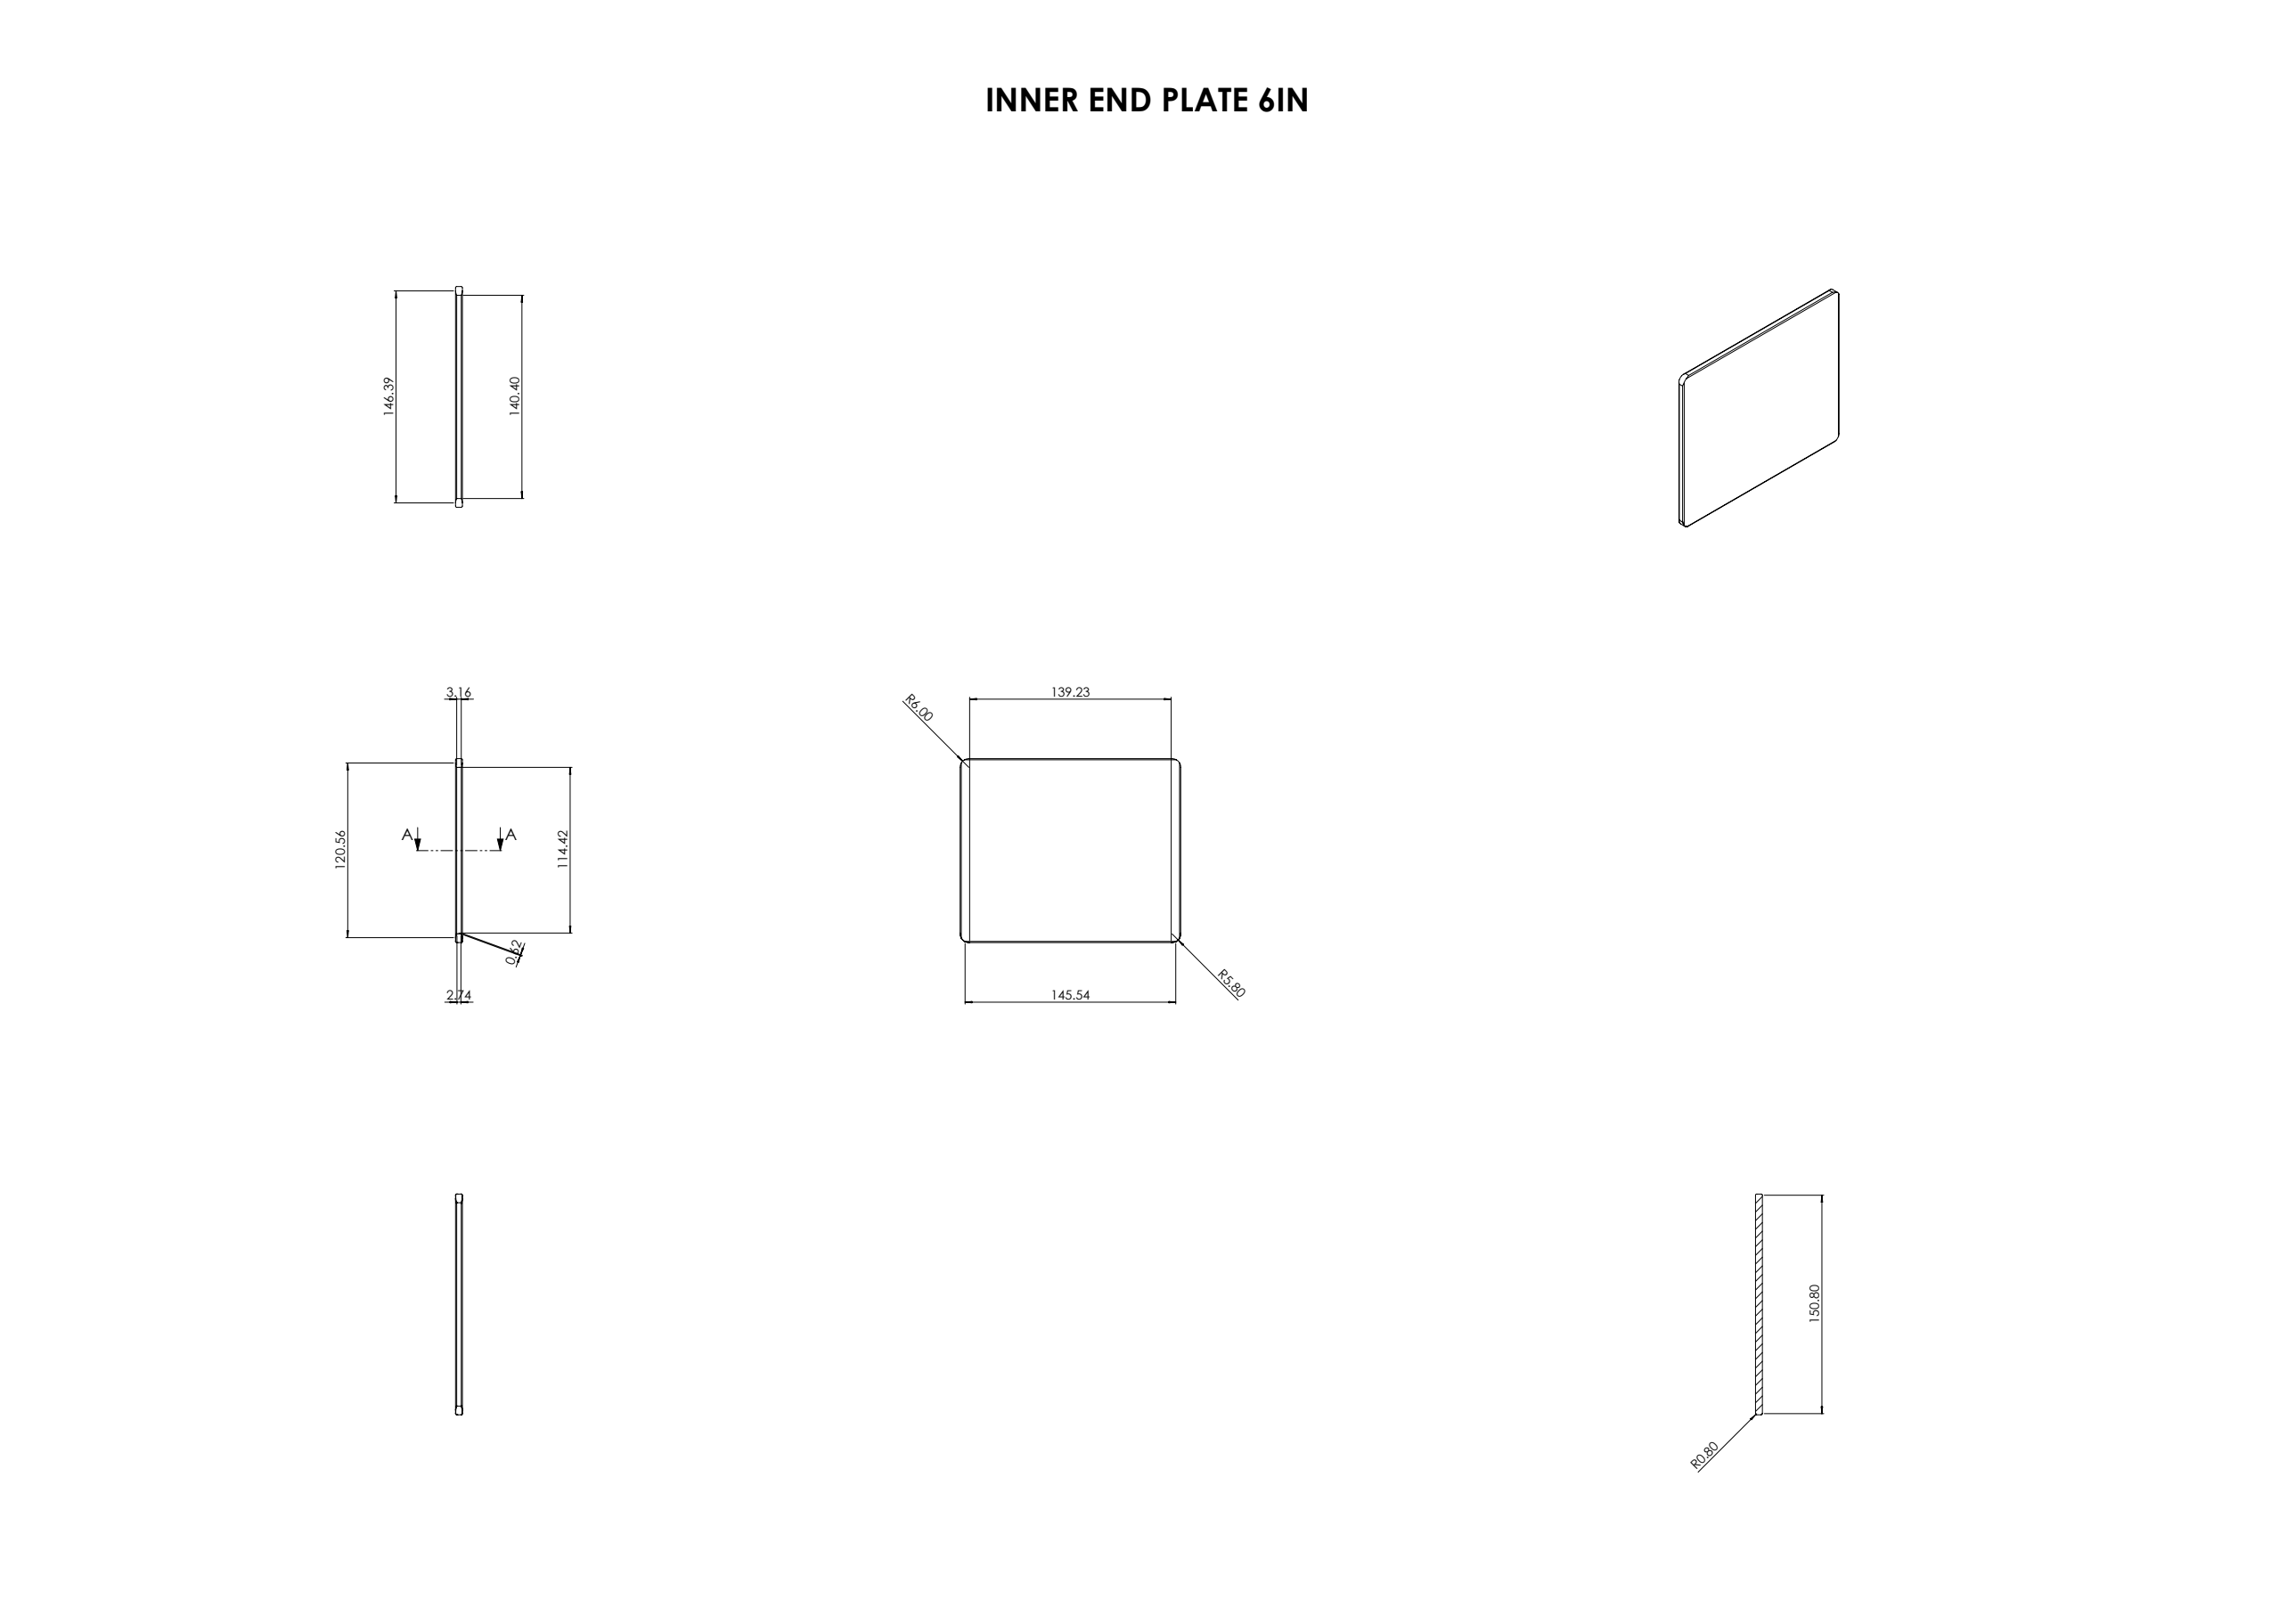
ISO-10303-21;
HEADER;
/* Generated by software containing ST-Developer
 * from STEP Tools, Inc. (www.steptools.com) 
 */

FILE_DESCRIPTION(
/* description */ (''),
/* implementation_level */ '2;1');

FILE_NAME(
/* name */ '06_Inner_End_Plate_6in.step',
/* time_stamp */ '2026-10-25T01:30:15-07:00',
/* author */ (''),
/* organization */ (''),
/* preprocessor_version */ 'ST-DEVELOPER v20.2',
/* originating_system */ 'Autodesk Translation Framework v15.15.0.0',
/* authorisation */ '');

FILE_SCHEMA (('AUTOMOTIVE_DESIGN { 1 0 10303 214 3 1 1 }'));
ENDSEC;

DATA;
#10=MECHANICAL_DESIGN_GEOMETRIC_PRESENTATION_REPRESENTATION('',(#568),#32309);
#192=B_SPLINE_CURVE_WITH_KNOTS('',3,(#22664,#22665,#22666,#22667,#22668,
#22669,#22670,#22671,#22672,#22673,#22674,#22675,#22676,#22677,#22678,#22679,
#22680,#22681,#22682,#22683,#22684,#22685,#22686,#22687,#22688,#22689,#22690,
#22691,#22692,#22693,#22694,#22695,#22696,#22697,#22698,#22699,#22700,#22701,
#22702,#22703,#22704,#22705,#22706,#22707,#22708,#22709,#22710,#22711,#22712,
#22713,#22714,#22715,#22716,#22717,#22718,#22719,#22720,#22721,#22722,#22723,
#22724,#22725,#22726,#22727,#22728,#22729,#22730,#22731,#22732,#22733,#22734,
#22735,#22736,#22737,#22738,#22739,#22740,#22741,#22742,#22743,#22744,#22745),
 .UNSPECIFIED.,.F.,.F.,(4,3,3,3,3,3,3,3,3,3,3,3,3,3,3,3,3,3,3,3,3,3,3,3,
3,3,3,4),(0.,0.0295705059221788,0.060515948666938,0.0926038162611793,0.126139587094163,
0.161619668951817,0.19997110704497,0.243460414557959,0.310976439008441,
0.354040411570413,0.394412885847263,0.429686039983613,0.462833624459996,
0.494651028940637,0.527129557033639,0.560643519237532,0.596019929716605,
0.634095033607031,0.676984117127751,0.757738087845813,0.799051738230702,
0.836280906722732,0.871099048170047,0.903485294449899,0.934889313351429,
0.965468174714213,0.9950913281628,1.),.UNSPECIFIED.);
#193=B_SPLINE_CURVE_WITH_KNOTS('',3,(#22747,#22748,#22749,#22750),
 .UNSPECIFIED.,.F.,.F.,(4,4),(-1.,0.),.UNSPECIFIED.);
#194=B_SPLINE_CURVE_WITH_KNOTS('',3,(#22752,#22753,#22754,#22755,#22756,
#22757,#22758,#22759,#22760,#22761,#22762,#22763,#22764,#22765,#22766,#22767,
#22768,#22769,#22770,#22771,#22772,#22773,#22774,#22775,#22776,#22777,#22778,
#22779,#22780,#22781,#22782,#22783,#22784,#22785,#22786,#22787,#22788,#22789,
#22790,#22791,#22792,#22793,#22794,#22795,#22796,#22797,#22798,#22799,#22800,
#22801,#22802,#22803),.UNSPECIFIED.,.F.,.F.,(4,3,3,3,3,3,3,3,3,3,3,3,3,
3,3,3,3,4),(0.,0.0499444622912523,0.102213229602865,0.161337747228745,0.226027789144595,
0.322774315501521,0.388018395848048,0.444871194111793,0.498045969161039,
0.55130803854745,0.608971254047864,0.676370635210691,0.757277976408018,
0.819640075218638,0.876287936111095,0.929442920609184,0.979183148027167,
1.),.UNSPECIFIED.);
#195=B_SPLINE_CURVE_WITH_KNOTS('',3,(#22843,#22844,#22845,#22846,#22847,
#22848,#22849,#22850,#22851,#22852,#22853,#22854,#22855,#22856,#22857,#22858,
#22859,#22860,#22861,#22862,#22863,#22864,#22865,#22866,#22867,#22868,#22869,
#22870,#22871,#22872,#22873,#22874,#22875,#22876,#22877,#22878,#22879,#22880,
#22881,#22882,#22883,#22884,#22885,#22886,#22887,#22888,#22889,#22890,#22891,
#22892,#22893,#22894),.UNSPECIFIED.,.F.,.F.,(4,3,3,3,3,3,3,3,3,3,3,3,3,
3,3,3,3,4),(0.,0.0499441826810774,0.102212661913948,0.161336812389012,0.22602629684231,
0.322773009737021,0.388016976561433,0.444869601982627,0.498043895325567,
0.551305755159732,0.608968423870093,0.676366592453384,0.757274944340038,
0.819637084908965,0.876284880238144,0.929439762109144,0.979179823244059,
1.),.UNSPECIFIED.);
#196=B_SPLINE_CURVE_WITH_KNOTS('',3,(#22896,#22897,#22898,#22899),
 .UNSPECIFIED.,.F.,.F.,(4,4),(0.,1.),.UNSPECIFIED.);
#197=B_SPLINE_CURVE_WITH_KNOTS('',3,(#22901,#22902,#22903,#22904,#22905,
#22906,#22907,#22908,#22909,#22910,#22911,#22912,#22913,#22914,#22915,#22916,
#22917,#22918,#22919,#22920,#22921,#22922,#22923,#22924,#22925,#22926,#22927,
#22928,#22929,#22930,#22931,#22932,#22933,#22934,#22935,#22936,#22937,#22938,
#22939,#22940,#22941,#22942,#22943,#22944,#22945,#22946,#22947,#22948,#22949,
#22950,#22951,#22952,#22953,#22954,#22955,#22956,#22957,#22958,#22959,#22960,
#22961,#22962,#22963,#22964,#22965,#22966,#22967,#22968,#22969,#22970,#22971,
#22972,#22973,#22974,#22975,#22976,#22977,#22978,#22979,#22980,#22981,#22982),
 .UNSPECIFIED.,.F.,.F.,(4,3,3,3,3,3,3,3,3,3,3,3,3,3,3,3,3,3,3,3,3,3,3,3,
3,3,3,4),(0.,0.0295773881145616,0.060530416968692,0.0926266479896254,0.126171922797507,
0.161663359409179,0.200029752326511,0.243548698803929,0.310961877352299,
0.35402676001778,0.394400087516669,0.429679984519188,0.462839399605369,
0.494661354038637,0.527132669662275,0.560640871657354,0.59601115409547,
0.63407950773062,0.676959315385358,0.757719486539019,0.799022960212248,
0.836244253893979,0.871055469575998,0.903435210203506,0.934833075272902,
0.965406057017476,0.995023142061764,1.),.UNSPECIFIED.);
#198=B_SPLINE_CURVE_WITH_KNOTS('',3,(#23001,#23002,#23003,#23004),
 .UNSPECIFIED.,.F.,.F.,(4,4),(9.99629094513139E-5,0.273153287835102),
 .UNSPECIFIED.);
#199=B_SPLINE_CURVE_WITH_KNOTS('',3,(#23007,#23008,#23009,#23010),
 .UNSPECIFIED.,.F.,.F.,(4,4),(-0.273153287835102,-9.99629094513139E-5),
 .UNSPECIFIED.);
#200=B_SPLINE_CURVE_WITH_KNOTS('',3,(#23036,#23037,#23038,#23039),
 .UNSPECIFIED.,.F.,.F.,(4,4),(-0.310482170393536,-0.273153287835088),
 .UNSPECIFIED.);
#201=B_SPLINE_CURVE_WITH_KNOTS('',3,(#23040,#23041,#23042,#23043),
 .UNSPECIFIED.,.F.,.F.,(4,4),(0.273153287835088,0.310482170393536),
 .UNSPECIFIED.);
#202=B_SPLINE_CURVE_WITH_KNOTS('',3,(#23069,#23070,#23071,#23072,#23073,
#23074),.UNSPECIFIED.,.F.,.F.,(4,2,4),(-0.954291288267866,-0.799150016166134,
-0.681237813527804),.UNSPECIFIED.);
#203=B_SPLINE_CURVE_WITH_KNOTS('',3,(#23077,#23078,#23079,#23080,#23081,
#23082),.UNSPECIFIED.,.F.,.F.,(4,2,4),(0.681237813527804,0.799150016166134,
0.954291288267866),.UNSPECIFIED.);
#204=B_SPLINE_CURVE_WITH_KNOTS('',3,(#23099,#23100,#23101,#23102),
 .UNSPECIFIED.,.F.,.F.,(4,4),(-0.681237813527818,-0.643908930969367),
 .UNSPECIFIED.);
#205=B_SPLINE_CURVE_WITH_KNOTS('',3,(#23103,#23104,#23105,#23106),
 .UNSPECIFIED.,.F.,.F.,(4,4),(0.643908930969367,0.681237813527818),
 .UNSPECIFIED.);
#206=B_SPLINE_CURVE_WITH_KNOTS('',3,(#23111,#23112,#23113,#23114,#23115,
#23116),.UNSPECIFIED.,.F.,.F.,(4,2,4),(0.,0.155241085196768,0.310482170393536),
 .UNSPECIFIED.);
#207=B_SPLINE_CURVE_WITH_KNOTS('',3,(#23130,#23131,#23132,#23133,#23134,
#23135,#23136,#23137,#23138,#23139,#23140,#23141,#23142,#23143,#23144,#23145,
#23146,#23147,#23148,#23149,#23150,#23151,#23152,#23153,#23154,#23155,#23156,
#23157,#23158,#23159,#23160,#23161,#23162,#23163,#23164,#23165,#23166,#23167,
#23168,#23169,#23170,#23171,#23172,#23173,#23174,#23175,#23176,#23177,#23178,
#23179,#23180,#23181),.UNSPECIFIED.,.F.,.F.,(4,3,3,3,3,3,3,3,3,3,3,3,3,
3,3,3,3,4),(0.,0.0499444619143997,0.102213228836067,0.161337745961679,0.226027787112555,
0.322774313723485,0.388018393939231,0.444871191980803,0.498045966386616,
0.551308035462484,0.608971250191218,0.676370629650621,0.757277972237966,
0.819640071099801,0.876287931893757,0.929442916241627,0.979183143421037,
1.),.UNSPECIFIED.);
#208=B_SPLINE_CURVE_WITH_KNOTS('',3,(#23183,#23184,#23185,#23186),
 .UNSPECIFIED.,.F.,.F.,(4,4),(0.681229980645393,0.954283455385461),
 .UNSPECIFIED.);
#209=B_SPLINE_CURVE_WITH_KNOTS('',3,(#23188,#23189,#23190,#23191),
 .UNSPECIFIED.,.F.,.F.,(4,4),(0.64390109808696,0.681229980645406),
 .UNSPECIFIED.);
#210=B_SPLINE_CURVE_WITH_KNOTS('',3,(#23195,#23196,#23197,#23198),
 .UNSPECIFIED.,.F.,.F.,(4,4),(0.273153287835084,0.310482170393536),
 .UNSPECIFIED.);
#211=B_SPLINE_CURVE_WITH_KNOTS('',3,(#23200,#23201,#23202,#23203),
 .UNSPECIFIED.,.F.,.F.,(4,4),(9.9962909451316E-5,0.273153287835098),
 .UNSPECIFIED.);
#212=B_SPLINE_CURVE_WITH_KNOTS('',3,(#23204,#23205,#23206,#23207,#23208,
#23209,#23210,#23211,#23212,#23213,#23214,#23215,#23216,#23217,#23218,#23219,
#23220,#23221,#23222,#23223,#23224,#23225,#23226,#23227,#23228,#23229,#23230,
#23231,#23232,#23233,#23234,#23235,#23236,#23237,#23238,#23239,#23240,#23241,
#23242,#23243,#23244,#23245,#23246,#23247,#23248,#23249,#23250,#23251,#23252,
#23253,#23254,#23255),.UNSPECIFIED.,.F.,.F.,(4,3,3,3,3,3,3,3,3,3,3,3,3,
3,3,3,3,4),(0.,0.0499441833890994,0.102212663354842,0.161336814770156,0.226026300658892,
0.322773013076531,0.388016980146127,0.44486960598537,0.498043900535783,
0.551305760953592,0.608968431113942,0.676366602895863,0.757274952171898,
0.819637092644225,0.876284888158664,0.929439770311992,0.979179831894635,
1.),.UNSPECIFIED.);
#213=B_SPLINE_CURVE_WITH_KNOTS('',3,(#23278,#23279,#23280,#23281,#23282,
#23283,#23284,#23285,#23286,#23287,#23288,#23289,#23290,#23291,#23292,#23293,
#23294,#23295,#23296,#23297,#23298,#23299,#23300,#23301,#23302,#23303,#23304,
#23305,#23306,#23307,#23308,#23309,#23310,#23311,#23312,#23313,#23314,#23315,
#23316,#23317,#23318,#23319,#23320,#23321,#23322,#23323,#23324,#23325,#23326,
#23327,#23328,#23329,#23330,#23331,#23332,#23333,#23334,#23335,#23336,#23337,
#23338,#23339,#23340,#23341,#23342,#23343,#23344,#23345,#23346,#23347,#23348,
#23349,#23350,#23351,#23352,#23353,#23354,#23355,#23356,#23357,#23358,#23359),
 .UNSPECIFIED.,.F.,.F.,(4,3,3,3,3,3,3,3,3,3,3,3,3,3,3,3,3,3,3,3,3,3,3,3,
3,3,3,4),(0.,0.0295705059449982,0.0605159487132195,0.0926038163323903,0.126139587195106,
0.161619669086869,0.199971107221821,0.243460414815925,0.310976439628805,
0.354040412152005,0.394412886392504,0.42968604051999,0.462833625082738,
0.494651029536218,0.527129557597107,0.56064351985676,0.596019930404549,
0.634095034387078,0.676984118085056,0.757738088563792,0.79905173888368,
0.836280907354532,0.871099048793566,0.903485295079146,0.934889313990762,
0.965468175362615,0.99509132882554,1.),.UNSPECIFIED.);
#214=B_SPLINE_CURVE_WITH_KNOTS('',3,(#23361,#23362,#23363,#23364),
 .UNSPECIFIED.,.F.,.F.,(4,4),(-1.,0.),.UNSPECIFIED.);
#215=B_SPLINE_CURVE_WITH_KNOTS('',3,(#23366,#23367,#23368,#23369,#23370,
#23371,#23372,#23373,#23374,#23375,#23376,#23377,#23378,#23379,#23380,#23381,
#23382,#23383,#23384,#23385,#23386,#23387,#23388,#23389,#23390,#23391,#23392,
#23393,#23394,#23395,#23396,#23397,#23398,#23399,#23400,#23401,#23402,#23403,
#23404,#23405,#23406,#23407,#23408,#23409,#23410,#23411,#23412,#23413,#23414,
#23415,#23416,#23417),.UNSPECIFIED.,.F.,.F.,(4,3,3,3,3,3,3,3,3,3,3,3,3,
3,3,3,3,4),(0.,0.0499444620030573,0.102213229017714,0.161337746261311,0.226027787592192,
0.322774314143168,0.388018394389041,0.444871192483061,0.498045967040621,
0.551308036189455,0.608971251099731,0.676370630959906,0.757277973219929,
0.819640072069571,0.876287932886441,0.929442917270342,0.979183144505862,
1.),.UNSPECIFIED.);
#216=B_SPLINE_CURVE_WITH_KNOTS('',3,(#23457,#23458,#23459,#23460,#23461,
#23462,#23463,#23464,#23465,#23466,#23467,#23468,#23469,#23470,#23471,#23472,
#23473,#23474,#23475,#23476,#23477,#23478,#23479,#23480,#23481,#23482,#23483,
#23484,#23485,#23486,#23487,#23488,#23489,#23490,#23491,#23492,#23493,#23494,
#23495,#23496,#23497,#23498,#23499,#23500,#23501,#23502,#23503,#23504,#23505,
#23506,#23507,#23508),.UNSPECIFIED.,.F.,.F.,(4,3,3,3,3,3,3,3,3,3,3,3,3,
3,3,3,3,4),(0.,0.0499441826811105,0.102212661914011,0.161336812389129,0.226026296842565,
0.322773009737244,0.388016976561584,0.444869601982792,0.498043895325763,
0.551305755159944,0.608968423870338,0.676366592453702,0.757274944340276,
0.819637084909205,0.876284880238396,0.929439762109376,0.979179823244325,
1.),.UNSPECIFIED.);
#217=B_SPLINE_CURVE_WITH_KNOTS('',3,(#23510,#23511,#23512,#23513),
 .UNSPECIFIED.,.F.,.F.,(4,4),(0.,1.),.UNSPECIFIED.);
#218=B_SPLINE_CURVE_WITH_KNOTS('',3,(#23515,#23516,#23517,#23518,#23519,
#23520,#23521,#23522,#23523,#23524,#23525,#23526,#23527,#23528,#23529,#23530,
#23531,#23532,#23533,#23534,#23535,#23536,#23537,#23538,#23539,#23540,#23541,
#23542,#23543,#23544,#23545,#23546,#23547,#23548,#23549,#23550,#23551,#23552,
#23553,#23554,#23555,#23556,#23557,#23558,#23559,#23560,#23561,#23562,#23563,
#23564,#23565,#23566,#23567,#23568,#23569,#23570,#23571,#23572,#23573,#23574,
#23575,#23576,#23577,#23578,#23579,#23580,#23581,#23582,#23583,#23584,#23585,
#23586,#23587,#23588,#23589,#23590,#23591,#23592,#23593,#23594,#23595,#23596),
 .UNSPECIFIED.,.F.,.F.,(4,3,3,3,3,3,3,3,3,3,3,3,3,3,3,3,3,3,3,3,3,3,3,3,
3,3,3,4),(0.,0.0295773881131102,0.0605304169672427,0.0926266479882803,0.126171922795967,
0.161663359407986,0.20002975232552,0.243548698802509,0.31096187735372,0.354026760019112,
0.394400087517918,0.429679984520021,0.462839399606215,0.494661354039968,
0.527132669663605,0.560640871658796,0.596011154096698,0.63407950773218,
0.676959315385293,0.75771948653897,0.799022960211628,0.836244253893244,
0.871055469575763,0.903435210203173,0.934833075272608,0.965406057016351,
0.995023142060179,1.),.UNSPECIFIED.);
#219=B_SPLINE_CURVE_WITH_KNOTS('',3,(#23615,#23616,#23617,#23618),
 .UNSPECIFIED.,.F.,.F.,(4,4),(9.99629094513149E-5,0.273153287835104),
 .UNSPECIFIED.);
#220=B_SPLINE_CURVE_WITH_KNOTS('',3,(#23621,#23622,#23623,#23624),
 .UNSPECIFIED.,.F.,.F.,(4,4),(-0.273153287835104,-9.99629094513149E-5),
 .UNSPECIFIED.);
#221=B_SPLINE_CURVE_WITH_KNOTS('',3,(#23650,#23651,#23652,#23653),
 .UNSPECIFIED.,.F.,.F.,(4,4),(-0.310482170393536,-0.273153287835091),
 .UNSPECIFIED.);
#222=B_SPLINE_CURVE_WITH_KNOTS('',3,(#23654,#23655,#23656,#23657),
 .UNSPECIFIED.,.F.,.F.,(4,4),(0.273153287835091,0.310482170393536),
 .UNSPECIFIED.);
#223=B_SPLINE_CURVE_WITH_KNOTS('',3,(#23675,#23676,#23677,#23678),
 .UNSPECIFIED.,.F.,.F.,(4,4),(-0.954283455385459,-0.681229980645392),
 .UNSPECIFIED.);
#224=B_SPLINE_CURVE_WITH_KNOTS('',3,(#23681,#23682,#23683,#23684),
 .UNSPECIFIED.,.F.,.F.,(4,4),(0.681229980645392,0.954283455385459),
 .UNSPECIFIED.);
#225=B_SPLINE_CURVE_WITH_KNOTS('',3,(#23701,#23702,#23703,#23704),
 .UNSPECIFIED.,.F.,.F.,(4,4),(-0.681229980645406,-0.643901098086959),
 .UNSPECIFIED.);
#226=B_SPLINE_CURVE_WITH_KNOTS('',3,(#23705,#23706,#23707,#23708),
 .UNSPECIFIED.,.F.,.F.,(4,4),(0.643901098086959,0.681229980645406),
 .UNSPECIFIED.);
#227=B_SPLINE_CURVE_WITH_KNOTS('',3,(#23722,#23723,#23724,#23725,#23726,
#23727),.UNSPECIFIED.,.F.,.F.,(4,2,4),(0.643901098086957,0.799142183283726,
0.954383268480494),.UNSPECIFIED.);
#228=B_SPLINE_CURVE_WITH_KNOTS('',3,(#23757,#23758,#23759,#23760,#23761,
#23762,#23763,#23764,#23765,#23766,#23767,#23768,#23769,#23770,#23771,#23772,
#23773,#23774,#23775,#23776,#23777,#23778,#23779,#23780,#23781,#23782,#23783,
#23784,#23785,#23786,#23787,#23788,#23789,#23790,#23791,#23792,#23793,#23794,
#23795,#23796,#23797,#23798,#23799,#23800,#23801,#23802,#23803,#23804,#23805,
#23806,#23807,#23808,#23809,#23810,#23811,#23812,#23813,#23814,#23815,#23816,
#23817,#23818,#23819,#23820,#23821,#23822,#23823,#23824,#23825,#23826,#23827,
#23828,#23829,#23830,#23831,#23832,#23833,#23834,#23835,#23836,#23837,#23838),
 .UNSPECIFIED.,.F.,.F.,(4,3,3,3,3,3,3,3,3,3,3,3,3,3,3,3,3,3,3,3,3,3,3,3,
3,3,3,4),(0.,0.0295705059512633,0.0605159487271851,0.0926038163550416,0.126139587225611,
0.161619669126796,0.199971107275455,0.243460414898968,0.31097643981881,
0.354040412330134,0.394412886559501,0.429686040686443,0.46283362527423,
0.494651029717672,0.527129557769278,0.560643520045596,0.596019930614712,
0.634095034624437,0.676984118378702,0.757738088784027,0.799051739082071,
0.836280907545797,0.871099048983326,0.903485295270873,0.934889314183803,
0.965468175561812,0.995091329030122,1.),.UNSPECIFIED.);
#229=B_SPLINE_CURVE_WITH_KNOTS('',3,(#23839,#23840,#23841,#23842),
 .UNSPECIFIED.,.F.,.F.,(4,4),(-1.,0.),.UNSPECIFIED.);
#230=B_SPLINE_CURVE_WITH_KNOTS('',3,(#23881,#23882,#23883,#23884),
 .UNSPECIFIED.,.F.,.F.,(4,4),(0.,1.),.UNSPECIFIED.);
#231=B_SPLINE_CURVE_WITH_KNOTS('',3,(#23885,#23886,#23887,#23888,#23889,
#23890,#23891,#23892,#23893,#23894,#23895,#23896,#23897,#23898,#23899,#23900,
#23901,#23902,#23903,#23904,#23905,#23906,#23907,#23908,#23909,#23910,#23911,
#23912,#23913,#23914,#23915,#23916,#23917,#23918,#23919,#23920,#23921,#23922,
#23923,#23924,#23925,#23926,#23927,#23928,#23929,#23930,#23931,#23932,#23933,
#23934,#23935,#23936,#23937,#23938,#23939,#23940,#23941,#23942,#23943,#23944,
#23945,#23946,#23947,#23948,#23949,#23950,#23951,#23952,#23953,#23954,#23955,
#23956,#23957,#23958,#23959,#23960,#23961,#23962,#23963,#23964,#23965,#23966),
 .UNSPECIFIED.,.F.,.F.,(4,3,3,3,3,3,3,3,3,3,3,3,3,3,3,3,3,3,3,3,3,3,3,3,
3,3,3,4),(0.,0.0295773880524302,0.0605304168410243,0.092626647792498,0.126171922525243,
0.161663359050634,0.200029751864124,0.24354869819935,0.31096188049952,0.3540267629683,
0.394400090282781,0.429679987033957,0.462839402284777,0.494661356438073,
0.527132671762529,0.560640873794645,0.59601115629688,0.634079510052112,
0.676959318040989,0.757719488530741,0.799022961866045,0.836244255350966,
0.871055470885213,0.903435211410382,0.934833076388468,0.965406058048494,
0.995023143024151,1.),.UNSPECIFIED.);
#232=B_SPLINE_CURVE_WITH_KNOTS('',3,(#23985,#23986,#23987,#23988),
 .UNSPECIFIED.,.F.,.F.,(4,4),(-0.273153287835098,-9.9962909451316E-5),
 .UNSPECIFIED.);
#233=B_SPLINE_CURVE_WITH_KNOTS('',3,(#24011,#24012,#24013,#24014),
 .UNSPECIFIED.,.F.,.F.,(4,4),(-0.310482170393536,-0.273153287835084),
 .UNSPECIFIED.);
#234=B_SPLINE_CURVE_WITH_KNOTS('',3,(#24032,#24033,#24034,#24035),
 .UNSPECIFIED.,.F.,.F.,(4,4),(-0.954283455385461,-0.681229980645393),
 .UNSPECIFIED.);
#235=B_SPLINE_CURVE_WITH_KNOTS('',3,(#24053,#24054,#24055,#24056),
 .UNSPECIFIED.,.F.,.F.,(4,4),(-0.681229980645406,-0.64390109808696),
 .UNSPECIFIED.);
#236=B_SPLINE_CURVE_WITH_KNOTS('',3,(#24061,#24062,#24063,#24064,#24065,
#24066,#24067,#24068,#24069,#24070,#24071,#24072,#24073,#24074,#24075,#24076,
#24077,#24078,#24079,#24080,#24081,#24082,#24083,#24084,#24085,#24086,#24087,
#24088,#24089,#24090,#24091,#24092,#24093,#24094,#24095,#24096,#24097,#24098,
#24099,#24100,#24101,#24102,#24103,#24104,#24105,#24106,#24107,#24108,#24109,
#24110,#24111,#24112,#24113,#24114,#24115,#24116,#24117,#24118,#24119,#24120,
#24121,#24122,#24123,#24124,#24125,#24126,#24127,#24128,#24129,#24130,#24131,
#24132,#24133,#24134,#24135,#24136,#24137,#24138,#24139,#24140,#24141,#24142),
 .UNSPECIFIED.,.F.,.F.,(4,3,3,3,3,3,3,3,3,3,3,3,3,3,3,3,3,3,3,3,3,3,3,3,
3,3,3,4),(0.,0.029577388096564,0.0605304169342327,0.092626647938075,0.126171922726201,
0.161663359317722,0.200029752207105,0.243548698650945,0.310961878143349,
0.354026760759389,0.394400088211927,0.42967998515154,0.462839400279756,
0.49466135464192,0.527132670190963,0.560640872195637,0.596011154650127,
0.634079508317272,0.676959316055784,0.757719487041838,0.799022960628449,
0.836244254262571,0.871055469905186,0.903435210506207,0.934833075552335,
0.965406057277606,0.995023142305148,1.),.UNSPECIFIED.);
#237=B_SPLINE_CURVE_WITH_KNOTS('',3,(#24144,#24145,#24146,#24147),
 .UNSPECIFIED.,.F.,.F.,(4,4),(-0.273153287835103,-9.99629094513129E-5),
 .UNSPECIFIED.);
#238=B_SPLINE_CURVE_WITH_KNOTS('',3,(#24175,#24176,#24177,#24178,#24179,
#24180,#24181,#24182,#24183,#24184,#24185,#24186,#24187,#24188,#24189,#24190,
#24191,#24192,#24193,#24194,#24195,#24196,#24197,#24198,#24199,#24200,#24201,
#24202,#24203,#24204,#24205,#24206,#24207,#24208,#24209,#24210,#24211,#24212,
#24213,#24214,#24215,#24216,#24217,#24218,#24219,#24220,#24221,#24222,#24223,
#24224,#24225,#24226,#24227,#24228,#24229,#24230,#24231,#24232,#24233,#24234,
#24235,#24236,#24237,#24238,#24239,#24240,#24241,#24242,#24243,#24244,#24245,
#24246,#24247,#24248,#24249,#24250,#24251,#24252,#24253,#24254,#24255,#24256),
 .UNSPECIFIED.,.F.,.F.,(4,3,3,3,3,3,3,3,3,3,3,3,3,3,3,3,3,3,3,3,3,3,3,3,
3,3,3,4),(0.,0.0295705059230571,0.0605159486675307,0.0926038162612098,0.126139587094081,
0.161619668951887,0.199971107044072,0.243460414557264,0.310976439007079,
0.354040411569137,0.394412885846066,0.429686039982072,0.462833624458263,
0.494651028937512,0.527129557030697,0.560643519234331,0.596019929713393,
0.634095033602269,0.676984117126932,0.757738087845199,0.799051738231756,
0.836280906723594,0.871099048170336,0.903485294450174,0.934889313352345,
0.965468174717861,0.99509132816655,1.),.UNSPECIFIED.);
#239=B_SPLINE_CURVE_WITH_KNOTS('',3,(#24258,#24259,#24260,#24261),
 .UNSPECIFIED.,.F.,.F.,(4,4),(-1.,0.),.UNSPECIFIED.);
#240=B_SPLINE_CURVE_WITH_KNOTS('',3,(#24262,#24263,#24264,#24265,#24266,
#24267,#24268,#24269,#24270,#24271,#24272,#24273,#24274,#24275,#24276,#24277,
#24278,#24279,#24280,#24281,#24282,#24283,#24284,#24285,#24286,#24287,#24288,
#24289,#24290,#24291,#24292,#24293,#24294,#24295,#24296,#24297,#24298,#24299,
#24300,#24301,#24302,#24303,#24304,#24305,#24306,#24307,#24308,#24309,#24310,
#24311,#24312,#24313),.UNSPECIFIED.,.F.,.F.,(4,3,3,3,3,3,3,3,3,3,3,3,3,
3,3,3,3,4),(0.,0.0499444622913127,0.102213229603,0.161337747229144,0.226027789144532,
0.322774315501466,0.388018395848148,0.444871194112166,0.498045969161075,
0.551308038547837,0.60897125404869,0.676370635211665,0.757277976408749,
0.81964007521899,0.876287936111462,0.92944292060967,0.979183148027608,1.),
 .UNSPECIFIED.);
#241=B_SPLINE_CURVE_WITH_KNOTS('',3,(#24351,#24352,#24353,#24354,#24355,
#24356,#24357,#24358,#24359,#24360,#24361,#24362,#24363,#24364,#24365,#24366,
#24367,#24368,#24369,#24370,#24371,#24372,#24373,#24374,#24375,#24376,#24377,
#24378,#24379,#24380,#24381,#24382,#24383,#24384,#24385,#24386,#24387,#24388,
#24389,#24390,#24391,#24392,#24393,#24394,#24395,#24396,#24397,#24398,#24399,
#24400,#24401,#24402),.UNSPECIFIED.,.F.,.F.,(4,3,3,3,3,3,3,3,3,3,3,3,3,
3,3,3,3,4),(0.,0.0499441828589668,0.102212662275513,0.161336812986304,0.226026297799104,
0.322773010574216,0.388016977460993,0.444869602986684,0.498043896631638,
0.551305756611869,0.608968425686129,0.676366595071555,0.757274946303666,
0.819637086848271,0.876284882223587,0.929439764165566,0.979179825412561,
1.),.UNSPECIFIED.);
#242=B_SPLINE_CURVE_WITH_KNOTS('',3,(#24403,#24404,#24405,#24406),
 .UNSPECIFIED.,.F.,.F.,(4,4),(0.,1.),.UNSPECIFIED.);
#243=B_SPLINE_CURVE_WITH_KNOTS('',3,(#24424,#24425,#24426,#24427),
 .UNSPECIFIED.,.F.,.F.,(4,4),(9.99629094513129E-5,0.273153287835103),
 .UNSPECIFIED.);
#244=B_SPLINE_CURVE_WITH_KNOTS('',3,(#24454,#24455,#24456,#24457),
 .UNSPECIFIED.,.F.,.F.,(4,4),(-0.310482170393537,-0.273153287835089),
 .UNSPECIFIED.);
#245=B_SPLINE_CURVE_WITH_KNOTS('',3,(#24458,#24459,#24460,#24461),
 .UNSPECIFIED.,.F.,.F.,(4,4),(0.273153287835089,0.310482170393537),
 .UNSPECIFIED.);
#246=B_SPLINE_CURVE_WITH_KNOTS('',3,(#24479,#24480,#24481,#24482),
 .UNSPECIFIED.,.F.,.F.,(4,4),(-0.95428345538546,-0.681229980645392),
 .UNSPECIFIED.);
#247=B_SPLINE_CURVE_WITH_KNOTS('',3,(#24485,#24486,#24487,#24488),
 .UNSPECIFIED.,.F.,.F.,(4,4),(0.681229980645392,0.95428345538546),
 .UNSPECIFIED.);
#248=B_SPLINE_CURVE_WITH_KNOTS('',3,(#24505,#24506,#24507,#24508),
 .UNSPECIFIED.,.F.,.F.,(4,4),(-0.681229980645405,-0.643901098086959),
 .UNSPECIFIED.);
#249=B_SPLINE_CURVE_WITH_KNOTS('',3,(#24509,#24510,#24511,#24512),
 .UNSPECIFIED.,.F.,.F.,(4,4),(0.643901098086959,0.681229980645405),
 .UNSPECIFIED.);
#250=B_SPLINE_CURVE_WITH_KNOTS('',3,(#24526,#24527,#24528,#24529,#24530,
#24531),.UNSPECIFIED.,.F.,.F.,(4,2,4),(0.,0.155241085196768,0.310482170393536),
 .UNSPECIFIED.);
#251=B_SPLINE_CURVE_WITH_KNOTS('',3,(#24534,#24535,#24536,#24537,#24538,
#24539),.UNSPECIFIED.,.F.,.F.,(4,2,4),(0.,0.155241085196768,0.310482170393535),
 .UNSPECIFIED.);
#252=B_SPLINE_CURVE_WITH_KNOTS('',3,(#24542,#24543,#24544,#24545,#24546,
#24547),.UNSPECIFIED.,.F.,.F.,(4,2,4),(0.643908930969365,0.799150016166132,
0.9543911013629),.UNSPECIFIED.);
#253=B_SPLINE_CURVE_WITH_KNOTS('',3,(#24550,#24551,#24552,#24553,#24554,
#24555),.UNSPECIFIED.,.F.,.F.,(4,2,4),(0.,0.15524108519677,0.310482170393539),
 .UNSPECIFIED.);
#254=B_SPLINE_CURVE_WITH_KNOTS('',3,(#24560,#24561,#24562,#24563,#24564,
#24565),.UNSPECIFIED.,.F.,.F.,(4,2,4),(0.643908930969368,0.799150016166137,
0.954391101362907),.UNSPECIFIED.);
#255=B_SPLINE_CURVE_WITH_KNOTS('',3,(#24566,#24567,#24568,#24569,#24570,
#24571),.UNSPECIFIED.,.F.,.F.,(4,2,4),(0.643908930969366,0.799150016166134,
0.954391101362902),.UNSPECIFIED.);
#447=B_SPLINE_SURFACE_WITH_KNOTS('',3,3,((#22642,#22643,#22644,#22645,#22646),
(#22647,#22648,#22649,#22650,#22651),(#22652,#22653,#22654,#22655,#22656),
(#22657,#22658,#22659,#22660,#22661)),.UNSPECIFIED.,.F.,.F.,.F.,(4,4),(4,
1,4),(0.,1.),(0.,0.571428571428571,1.),.UNSPECIFIED.);
#448=B_SPLINE_SURFACE_WITH_KNOTS('',3,3,((#22805,#22806,#22807,#22808,#22809,
#22810,#22811,#22812,#22813),(#22814,#22815,#22816,#22817,#22818,#22819,
#22820,#22821,#22822),(#22823,#22824,#22825,#22826,#22827,#22828,#22829,
#22830,#22831),(#22832,#22833,#22834,#22835,#22836,#22837,#22838,#22839,
#22840)),.UNSPECIFIED.,.F.,.F.,.F.,(4,4),(4,1,1,1,1,1,4),(0.,1.),(0.,0.214285714285714,
0.357142857142857,0.571428571428571,0.785714285714286,0.857142857142857,
1.),.UNSPECIFIED.);
#449=B_SPLINE_SURFACE_WITH_KNOTS('',3,3,((#22984,#22985,#22986,#22987),
(#22988,#22989,#22990,#22991),(#22992,#22993,#22994,#22995),(#22996,#22997,
#22998,#22999)),.UNSPECIFIED.,.F.,.F.,.F.,(4,4),(4,4),(0.,1.),(9.99629094513139E-5,
0.273153287835102),.UNSPECIFIED.);
#450=B_SPLINE_SURFACE_WITH_KNOTS('',3,3,((#23020,#23021,#23022,#23023),
(#23024,#23025,#23026,#23027),(#23028,#23029,#23030,#23031),(#23032,#23033,
#23034,#23035)),.UNSPECIFIED.,.F.,.F.,.F.,(4,4),(4,4),(0.,1.),(0.273153287835088,
0.310482170393536),.UNSPECIFIED.);
#451=B_SPLINE_SURFACE_WITH_KNOTS('',3,3,((#23044,#23045,#23046,#23047,#23048,
#23049),(#23050,#23051,#23052,#23053,#23054,#23055),(#23056,#23057,#23058,
#23059,#23060,#23061),(#23062,#23063,#23064,#23065,#23066,#23067)),
 .UNSPECIFIED.,.F.,.F.,.F.,(4,4),(4,2,4),(0.,1.),(0.681237813527804,0.799150016166134,
0.954291288267866),.UNSPECIFIED.);
#452=B_SPLINE_SURFACE_WITH_KNOTS('',3,3,((#23083,#23084,#23085,#23086),
(#23087,#23088,#23089,#23090),(#23091,#23092,#23093,#23094),(#23095,#23096,
#23097,#23098)),.UNSPECIFIED.,.F.,.F.,.F.,(4,4),(4,4),(0.,1.),(0.643908930969367,
0.681237813527818),.UNSPECIFIED.);
#453=B_SPLINE_SURFACE_WITH_KNOTS('',3,3,((#23256,#23257,#23258,#23259,#23260),
(#23261,#23262,#23263,#23264,#23265),(#23266,#23267,#23268,#23269,#23270),
(#23271,#23272,#23273,#23274,#23275)),.UNSPECIFIED.,.F.,.F.,.F.,(4,4),(4,
1,4),(0.,1.),(0.,0.571428571428571,1.),.UNSPECIFIED.);
#454=B_SPLINE_SURFACE_WITH_KNOTS('',3,3,((#23419,#23420,#23421,#23422,#23423,
#23424,#23425,#23426,#23427),(#23428,#23429,#23430,#23431,#23432,#23433,
#23434,#23435,#23436),(#23437,#23438,#23439,#23440,#23441,#23442,#23443,
#23444,#23445),(#23446,#23447,#23448,#23449,#23450,#23451,#23452,#23453,
#23454)),.UNSPECIFIED.,.F.,.F.,.F.,(4,4),(4,1,1,1,1,1,4),(0.,1.),(0.,0.214285714285714,
0.357142857142857,0.571428571428571,0.785714285714286,0.857142857142857,
1.),.UNSPECIFIED.);
#455=B_SPLINE_SURFACE_WITH_KNOTS('',3,3,((#23598,#23599,#23600,#23601),
(#23602,#23603,#23604,#23605),(#23606,#23607,#23608,#23609),(#23610,#23611,
#23612,#23613)),.UNSPECIFIED.,.F.,.F.,.F.,(4,4),(4,4),(0.,1.),(9.99629094513149E-5,
0.273153287835104),.UNSPECIFIED.);
#456=B_SPLINE_SURFACE_WITH_KNOTS('',3,3,((#23634,#23635,#23636,#23637),
(#23638,#23639,#23640,#23641),(#23642,#23643,#23644,#23645),(#23646,#23647,
#23648,#23649)),.UNSPECIFIED.,.F.,.F.,.F.,(4,4),(4,4),(0.,1.),(0.273153287835091,
0.310482170393536),.UNSPECIFIED.);
#457=B_SPLINE_SURFACE_WITH_KNOTS('',3,3,((#23658,#23659,#23660,#23661),
(#23662,#23663,#23664,#23665),(#23666,#23667,#23668,#23669),(#23670,#23671,
#23672,#23673)),.UNSPECIFIED.,.F.,.F.,.F.,(4,4),(4,4),(0.,1.),(0.681229980645392,
0.954283455385459),.UNSPECIFIED.);
#458=B_SPLINE_SURFACE_WITH_KNOTS('',3,3,((#23685,#23686,#23687,#23688),
(#23689,#23690,#23691,#23692),(#23693,#23694,#23695,#23696),(#23697,#23698,
#23699,#23700)),.UNSPECIFIED.,.F.,.F.,.F.,(4,4),(4,4),(0.,1.),(0.643901098086959,
0.681229980645406),.UNSPECIFIED.);
#459=B_SPLINE_SURFACE_WITH_KNOTS('',3,3,((#23735,#23736,#23737,#23738,#23739),
(#23740,#23741,#23742,#23743,#23744),(#23745,#23746,#23747,#23748,#23749),
(#23750,#23751,#23752,#23753,#23754)),.UNSPECIFIED.,.F.,.F.,.F.,(4,4),(4,
1,4),(0.,1.),(0.,0.571428571428571,1.),.UNSPECIFIED.);
#460=B_SPLINE_SURFACE_WITH_KNOTS('',3,3,((#23844,#23845,#23846,#23847,#23848,
#23849,#23850,#23851,#23852),(#23853,#23854,#23855,#23856,#23857,#23858,
#23859,#23860,#23861),(#23862,#23863,#23864,#23865,#23866,#23867,#23868,
#23869,#23870),(#23871,#23872,#23873,#23874,#23875,#23876,#23877,#23878,
#23879)),.UNSPECIFIED.,.F.,.F.,.F.,(4,4),(4,1,1,1,1,1,4),(0.,1.),(0.,0.214285714285714,
0.357142857142857,0.571428571428571,0.785714285714286,0.857142857142857,
1.),.UNSPECIFIED.);
#461=B_SPLINE_SURFACE_WITH_KNOTS('',3,3,((#23967,#23968,#23969,#23970),
(#23971,#23972,#23973,#23974),(#23975,#23976,#23977,#23978),(#23979,#23980,
#23981,#23982)),.UNSPECIFIED.,.F.,.F.,.F.,(4,4),(4,4),(0.,1.),(9.9962909451316E-5,
0.273153287835098),.UNSPECIFIED.);
#462=B_SPLINE_SURFACE_WITH_KNOTS('',3,3,((#23995,#23996,#23997,#23998),
(#23999,#24000,#24001,#24002),(#24003,#24004,#24005,#24006),(#24007,#24008,
#24009,#24010)),.UNSPECIFIED.,.F.,.F.,.F.,(4,4),(4,4),(0.,1.),(0.273153287835084,
0.310482170393536),.UNSPECIFIED.);
#463=B_SPLINE_SURFACE_WITH_KNOTS('',3,3,((#24015,#24016,#24017,#24018),
(#24019,#24020,#24021,#24022),(#24023,#24024,#24025,#24026),(#24027,#24028,
#24029,#24030)),.UNSPECIFIED.,.F.,.F.,.F.,(4,4),(4,4),(0.,1.),(0.681229980645393,
0.954283455385461),.UNSPECIFIED.);
#464=B_SPLINE_SURFACE_WITH_KNOTS('',3,3,((#24037,#24038,#24039,#24040),
(#24041,#24042,#24043,#24044),(#24045,#24046,#24047,#24048),(#24049,#24050,
#24051,#24052)),.UNSPECIFIED.,.F.,.F.,.F.,(4,4),(4,4),(0.,1.),(0.64390109808696,
0.681229980645406),.UNSPECIFIED.);
#465=B_SPLINE_SURFACE_WITH_KNOTS('',3,3,((#24154,#24155,#24156,#24157,#24158),
(#24159,#24160,#24161,#24162,#24163),(#24164,#24165,#24166,#24167,#24168),
(#24169,#24170,#24171,#24172,#24173)),.UNSPECIFIED.,.F.,.F.,.F.,(4,4),(4,
1,4),(0.,1.),(0.,0.571428571428571,1.),.UNSPECIFIED.);
#466=B_SPLINE_SURFACE_WITH_KNOTS('',3,3,((#24314,#24315,#24316,#24317,#24318,
#24319,#24320,#24321,#24322),(#24323,#24324,#24325,#24326,#24327,#24328,
#24329,#24330,#24331),(#24332,#24333,#24334,#24335,#24336,#24337,#24338,
#24339,#24340),(#24341,#24342,#24343,#24344,#24345,#24346,#24347,#24348,
#24349)),.UNSPECIFIED.,.F.,.F.,.F.,(4,4),(4,1,1,1,1,1,4),(0.,1.),(0.,0.214285714285714,
0.357142857142857,0.571428571428571,0.785714285714286,0.857142857142857,
1.),.UNSPECIFIED.);
#467=B_SPLINE_SURFACE_WITH_KNOTS('',3,3,((#24407,#24408,#24409,#24410),
(#24411,#24412,#24413,#24414),(#24415,#24416,#24417,#24418),(#24419,#24420,
#24421,#24422)),.UNSPECIFIED.,.F.,.F.,.F.,(4,4),(4,4),(0.,1.),(9.99629094513129E-5,
0.273153287835103),.UNSPECIFIED.);
#468=B_SPLINE_SURFACE_WITH_KNOTS('',3,3,((#24438,#24439,#24440,#24441),
(#24442,#24443,#24444,#24445),(#24446,#24447,#24448,#24449),(#24450,#24451,
#24452,#24453)),.UNSPECIFIED.,.F.,.F.,.F.,(4,4),(4,4),(0.,1.),(0.273153287835089,
0.310482170393537),.UNSPECIFIED.);
#469=B_SPLINE_SURFACE_WITH_KNOTS('',3,3,((#24462,#24463,#24464,#24465),
(#24466,#24467,#24468,#24469),(#24470,#24471,#24472,#24473),(#24474,#24475,
#24476,#24477)),.UNSPECIFIED.,.F.,.F.,.F.,(4,4),(4,4),(0.,1.),(0.681229980645392,
0.95428345538546),.UNSPECIFIED.);
#470=B_SPLINE_SURFACE_WITH_KNOTS('',3,3,((#24489,#24490,#24491,#24492),
(#24493,#24494,#24495,#24496),(#24497,#24498,#24499,#24500),(#24501,#24502,
#24503,#24504)),.UNSPECIFIED.,.F.,.F.,.F.,(4,4),(4,4),(0.,1.),(0.643901098086959,
0.681229980645405),.UNSPECIFIED.);
#540=SHAPE_REPRESENTATION_RELATIONSHIP('SRR','None',#32367,#554);
#554=ADVANCED_BREP_SHAPE_REPRESENTATION('',(#582),#32300);
#568=STYLED_ITEM('',(#32495),#582);
#582=MANIFOLD_SOLID_BREP('Body1',#13809);
#706=CYLINDRICAL_SURFACE('',#14382,0.8);
#707=CYLINDRICAL_SURFACE('',#14384,6.00000000000001);
#708=CYLINDRICAL_SURFACE('',#14390,0.8);
#709=CYLINDRICAL_SURFACE('',#14396,0.8);
#710=CYLINDRICAL_SURFACE('',#14404,6.00000000000001);
#711=CYLINDRICAL_SURFACE('',#14405,0.8);
#712=CYLINDRICAL_SURFACE('',#14406,0.8);
#713=CYLINDRICAL_SURFACE('',#14407,5.99999999999998);
#714=CYLINDRICAL_SURFACE('',#14408,0.8);
#715=CYLINDRICAL_SURFACE('',#14409,6.);
#716=CYLINDRICAL_SURFACE('',#14411,0.8);
#717=CYLINDRICAL_SURFACE('',#14412,0.8);
#939=CIRCLE('',#14380,5.80000000000001);
#940=CIRCLE('',#14381,6.00000000000001);
#941=CIRCLE('',#14385,6.00000000000001);
#942=CIRCLE('',#14387,5.80000000000001);
#943=CIRCLE('',#14388,6.00000000000001);
#944=CIRCLE('',#14392,6.);
#945=CIRCLE('',#14393,5.99999999999998);
#946=CIRCLE('',#14395,5.80000000000001);
#947=CIRCLE('',#14399,5.80000000000001);
#948=CIRCLE('',#14400,6.00000000000001);
#949=CIRCLE('',#14402,5.99999999999998);
#950=CIRCLE('',#14403,6.);
#1177=CONICAL_SURFACE('',#14379,5.90000000000001,0.785398163397448);
#1178=CONICAL_SURFACE('',#14386,5.90000000000001,0.785398163397451);
#1179=CONICAL_SURFACE('',#14394,5.90000000000001,0.785398163397448);
#1180=CONICAL_SURFACE('',#14398,5.90000000000001,0.785398163397451);
#1515=FACE_OUTER_BOUND('',#2350,.T.);
#1516=FACE_OUTER_BOUND('',#2351,.T.);
#1517=FACE_OUTER_BOUND('',#2352,.T.);
#1518=FACE_OUTER_BOUND('',#2353,.T.);
#1519=FACE_OUTER_BOUND('',#2354,.T.);
#1520=FACE_OUTER_BOUND('',#2355,.T.);
#1521=FACE_OUTER_BOUND('',#2356,.T.);
#1522=FACE_OUTER_BOUND('',#2357,.T.);
#1523=FACE_OUTER_BOUND('',#2358,.T.);
#1524=FACE_OUTER_BOUND('',#2359,.T.);
#1525=FACE_OUTER_BOUND('',#2360,.T.);
#1526=FACE_OUTER_BOUND('',#2361,.T.);
#1527=FACE_OUTER_BOUND('',#2362,.T.);
#1528=FACE_OUTER_BOUND('',#2363,.T.);
#1529=FACE_OUTER_BOUND('',#2364,.T.);
#1530=FACE_OUTER_BOUND('',#2365,.T.);
#1531=FACE_OUTER_BOUND('',#2366,.T.);
#1532=FACE_OUTER_BOUND('',#2367,.T.);
#1533=FACE_OUTER_BOUND('',#2368,.T.);
#1534=FACE_OUTER_BOUND('',#2369,.T.);
#1535=FACE_OUTER_BOUND('',#2370,.T.);
#1536=FACE_OUTER_BOUND('',#2371,.T.);
#1537=FACE_OUTER_BOUND('',#2372,.T.);
#1538=FACE_OUTER_BOUND('',#2373,.T.);
#1539=FACE_OUTER_BOUND('',#2374,.T.);
#1540=FACE_OUTER_BOUND('',#2375,.T.);
#1541=FACE_OUTER_BOUND('',#2376,.T.);
#1542=FACE_OUTER_BOUND('',#2377,.T.);
#1543=FACE_OUTER_BOUND('',#2378,.T.);
#1544=FACE_OUTER_BOUND('',#2379,.T.);
#1545=FACE_OUTER_BOUND('',#2380,.T.);
#1546=FACE_OUTER_BOUND('',#2381,.T.);
#1547=FACE_OUTER_BOUND('',#2382,.T.);
#1548=FACE_OUTER_BOUND('',#2383,.T.);
#1549=FACE_OUTER_BOUND('',#2384,.T.);
#1550=FACE_OUTER_BOUND('',#2385,.T.);
#1551=FACE_OUTER_BOUND('',#2386,.T.);
#1552=FACE_OUTER_BOUND('',#2387,.T.);
#1553=FACE_OUTER_BOUND('',#2388,.T.);
#1554=FACE_OUTER_BOUND('',#2389,.T.);
#1555=FACE_OUTER_BOUND('',#2390,.T.);
#1556=FACE_OUTER_BOUND('',#2391,.T.);
#1557=FACE_OUTER_BOUND('',#2392,.T.);
#1558=FACE_OUTER_BOUND('',#2393,.T.);
#1559=FACE_OUTER_BOUND('',#2394,.T.);
#1560=FACE_OUTER_BOUND('',#2395,.T.);
#2350=EDGE_LOOP('',(#9961,#9962,#9963,#9964));
#2351=EDGE_LOOP('',(#9965,#9966,#9967,#9968));
#2352=EDGE_LOOP('',(#9969,#9970,#9971,#9972));
#2353=EDGE_LOOP('',(#9973,#9974,#9975,#9976));
#2354=EDGE_LOOP('',(#9977,#9978,#9979,#9980));
#2355=EDGE_LOOP('',(#9981,#9982,#9983,#9984));
#2356=EDGE_LOOP('',(#9985,#9986,#9987,#9988));
#2357=EDGE_LOOP('',(#9989,#9990,#9991,#9992,#9993));
#2358=EDGE_LOOP('',(#9994,#9995,#9996,#9997,#9998,#9999));
#2359=EDGE_LOOP('',(#10000,#10001,#10002,#10003,#10004,#10005,#10006,#10007,
#10008,#10009,#10010,#10011,#10012,#10013,#10014,#10015));
#2360=EDGE_LOOP('',(#10016,#10017,#10018,#10019));
#2361=EDGE_LOOP('',(#10020,#10021,#10022,#10023));
#2362=EDGE_LOOP('',(#10024,#10025,#10026,#10027));
#2363=EDGE_LOOP('',(#10028,#10029,#10030,#10031));
#2364=EDGE_LOOP('',(#10032,#10033,#10034,#10035));
#2365=EDGE_LOOP('',(#10036,#10037,#10038,#10039));
#2366=EDGE_LOOP('',(#10040,#10041,#10042,#10043));
#2367=EDGE_LOOP('',(#10044,#10045,#10046,#10047,#10048,#10049));
#2368=EDGE_LOOP('',(#10050,#10051,#10052,#10053,#10054));
#2369=EDGE_LOOP('',(#10055,#10056,#10057,#10058,#10059,#10060,#10061,#10062,
#10063,#10064,#10065,#10066));
#2370=EDGE_LOOP('',(#10067,#10068,#10069,#10070));
#2371=EDGE_LOOP('',(#10071,#10072,#10073,#10074));
#2372=EDGE_LOOP('',(#10075,#10076,#10077,#10078));
#2373=EDGE_LOOP('',(#10079,#10080,#10081,#10082));
#2374=EDGE_LOOP('',(#10083,#10084,#10085,#10086));
#2375=EDGE_LOOP('',(#10087,#10088,#10089,#10090));
#2376=EDGE_LOOP('',(#10091,#10092,#10093,#10094));
#2377=EDGE_LOOP('',(#10095,#10096,#10097,#10098,#10099,#10100));
#2378=EDGE_LOOP('',(#10101,#10102,#10103,#10104,#10105,#10106,#10107,#10108));
#2379=EDGE_LOOP('',(#10109,#10110,#10111,#10112));
#2380=EDGE_LOOP('',(#10113,#10114,#10115,#10116));
#2381=EDGE_LOOP('',(#10117,#10118,#10119,#10120));
#2382=EDGE_LOOP('',(#10121,#10122,#10123,#10124));
#2383=EDGE_LOOP('',(#10125,#10126,#10127,#10128));
#2384=EDGE_LOOP('',(#10129,#10130,#10131,#10132));
#2385=EDGE_LOOP('',(#10133,#10134,#10135,#10136));
#2386=EDGE_LOOP('',(#10137,#10138,#10139,#10140,#10141,#10142,#10143,#10144,
#10145,#10146,#10147,#10148));
#2387=EDGE_LOOP('',(#10149,#10150,#10151,#10152,#10153,#10154,#10155,#10156,
#10157,#10158,#10159,#10160,#10161,#10162,#10163,#10164));
#2388=EDGE_LOOP('',(#10165,#10166,#10167,#10168,#10169,#10170));
#2389=EDGE_LOOP('',(#10171,#10172,#10173,#10174,#10175));
#2390=EDGE_LOOP('',(#10176,#10177,#10178,#10179,#10180,#10181,#10182,#10183));
#2391=EDGE_LOOP('',(#10184,#10185,#10186,#10187));
#2392=EDGE_LOOP('',(#10188,#10189,#10190,#10191,#10192,#10193,#10194,#10195));
#2393=EDGE_LOOP('',(#10196,#10197,#10198,#10199));
#2394=EDGE_LOOP('',(#10200,#10201,#10202,#10203));
#2395=EDGE_LOOP('',(#10204,#10205,#10206,#10207,#10208));
#3267=LINE('',#22804,#4578);
#3268=LINE('',#22983,#4579);
#3269=LINE('',#23006,#4580);
#3270=LINE('',#23014,#4581);
#3271=LINE('',#23018,#4582);
#3272=LINE('',#23076,#4583);
#3273=LINE('',#23109,#4584);
#3274=LINE('',#23117,#4585);
#3275=LINE('',#23120,#4586);
#3276=LINE('',#23122,#4587);
#3277=LINE('',#23124,#4588);
#3278=LINE('',#23125,#4589);
#3279=LINE('',#23128,#4590);
#3280=LINE('',#23418,#4591);
#3281=LINE('',#23597,#4592);
#3282=LINE('',#23620,#4593);
#3283=LINE('',#23628,#4594);
#3284=LINE('',#23632,#4595);
#3285=LINE('',#23680,#4596);
#3286=LINE('',#23711,#4597);
#3287=LINE('',#23713,#4598);
#3288=LINE('',#23715,#4599);
#3289=LINE('',#23717,#4600);
#3290=LINE('',#23718,#4601);
#3291=LINE('',#23721,#4602);
#3292=LINE('',#23732,#4603);
#3293=LINE('',#23734,#4604);
#3294=LINE('',#23843,#4605);
#3295=LINE('',#23984,#4606);
#3296=LINE('',#23991,#4607);
#3297=LINE('',#23994,#4608);
#3298=LINE('',#24036,#4609);
#3299=LINE('',#24059,#4610);
#3300=LINE('',#24148,#4611);
#3301=LINE('',#24150,#4612);
#3302=LINE('',#24152,#4613);
#3303=LINE('',#24153,#4614);
#3304=LINE('',#24428,#4615);
#3305=LINE('',#24432,#4616);
#3306=LINE('',#24436,#4617);
#3307=LINE('',#24484,#4618);
#3308=LINE('',#24515,#4619);
#3309=LINE('',#24519,#4620);
#3310=LINE('',#24522,#4621);
#3311=LINE('',#24541,#4622);
#3312=LINE('',#24556,#4623);
#3313=LINE('',#24559,#4624);
#3314=LINE('',#24573,#4625);
#4578=VECTOR('',#16187,10.);
#4579=VECTOR('',#16188,10.);
#4580=VECTOR('',#16189,10.);
#4581=VECTOR('',#16192,10.);
#4582=VECTOR('',#16195,10.);
#4583=VECTOR('',#16198,10.);
#4584=VECTOR('',#16201,10.);
#4585=VECTOR('',#16202,10.);
#4586=VECTOR('',#16205,10.);
#4587=VECTOR('',#16206,10.);
#4588=VECTOR('',#16207,10.);
#4589=VECTOR('',#16208,10.);
#4590=VECTOR('',#16211,10.);
#4591=VECTOR('',#16214,10.);
#4592=VECTOR('',#16215,10.);
#4593=VECTOR('',#16216,10.);
#4594=VECTOR('',#16219,10.);
#4595=VECTOR('',#16222,10.);
#4596=VECTOR('',#16225,10.);
#4597=VECTOR('',#16228,10.);
#4598=VECTOR('',#16229,10.);
#4599=VECTOR('',#16230,10.);
#4600=VECTOR('',#16231,10.);
#4601=VECTOR('',#16232,10.);
#4602=VECTOR('',#16235,10.);
#4603=VECTOR('',#16240,10.);
#4604=VECTOR('',#16243,10.);
#4605=VECTOR('',#16244,10.);
#4606=VECTOR('',#16245,10.);
#4607=VECTOR('',#16248,10.);
#4608=VECTOR('',#16251,10.);
#4609=VECTOR('',#16252,10.);
#4610=VECTOR('',#16255,10.);
#4611=VECTOR('',#16256,10.);
#4612=VECTOR('',#16259,10.);
#4613=VECTOR('',#16260,10.);
#4614=VECTOR('',#16261,10.);
#4615=VECTOR('',#16262,10.);
#4616=VECTOR('',#16265,10.);
#4617=VECTOR('',#16268,10.);
#4618=VECTOR('',#16271,10.);
#4619=VECTOR('',#16274,10.);
#4620=VECTOR('',#16277,10.);
#4621=VECTOR('',#16280,10.);
#4622=VECTOR('',#16289,10.);
#4623=VECTOR('',#16292,10.);
#4624=VECTOR('',#16295,10.);
#4625=VECTOR('',#16298,10.);
#5896=VERTEX_POINT('',#22662);
#5897=VERTEX_POINT('',#22663);
#5898=VERTEX_POINT('',#22746);
#5899=VERTEX_POINT('',#22751);
#5900=VERTEX_POINT('',#22841);
#5901=VERTEX_POINT('',#22842);
#5902=VERTEX_POINT('',#22895);
#5903=VERTEX_POINT('',#22900);
#5904=VERTEX_POINT('',#23000);
#5905=VERTEX_POINT('',#23005);
#5906=VERTEX_POINT('',#23012);
#5907=VERTEX_POINT('',#23013);
#5908=VERTEX_POINT('',#23015);
#5909=VERTEX_POINT('',#23017);
#5910=VERTEX_POINT('',#23068);
#5911=VERTEX_POINT('',#23075);
#5912=VERTEX_POINT('',#23108);
#5913=VERTEX_POINT('',#23110);
#5914=VERTEX_POINT('',#23119);
#5915=VERTEX_POINT('',#23121);
#5916=VERTEX_POINT('',#23123);
#5917=VERTEX_POINT('',#23127);
#5918=VERTEX_POINT('',#23129);
#5919=VERTEX_POINT('',#23182);
#5920=VERTEX_POINT('',#23187);
#5921=VERTEX_POINT('',#23192);
#5922=VERTEX_POINT('',#23194);
#5923=VERTEX_POINT('',#23199);
#5924=VERTEX_POINT('',#23276);
#5925=VERTEX_POINT('',#23277);
#5926=VERTEX_POINT('',#23360);
#5927=VERTEX_POINT('',#23365);
#5928=VERTEX_POINT('',#23455);
#5929=VERTEX_POINT('',#23456);
#5930=VERTEX_POINT('',#23509);
#5931=VERTEX_POINT('',#23514);
#5932=VERTEX_POINT('',#23614);
#5933=VERTEX_POINT('',#23619);
#5934=VERTEX_POINT('',#23626);
#5935=VERTEX_POINT('',#23627);
#5936=VERTEX_POINT('',#23629);
#5937=VERTEX_POINT('',#23631);
#5938=VERTEX_POINT('',#23674);
#5939=VERTEX_POINT('',#23679);
#5940=VERTEX_POINT('',#23710);
#5941=VERTEX_POINT('',#23712);
#5942=VERTEX_POINT('',#23714);
#5943=VERTEX_POINT('',#23716);
#5944=VERTEX_POINT('',#23720);
#5945=VERTEX_POINT('',#23729);
#5946=VERTEX_POINT('',#23731);
#5947=VERTEX_POINT('',#23755);
#5948=VERTEX_POINT('',#23756);
#5949=VERTEX_POINT('',#23880);
#5950=VERTEX_POINT('',#23983);
#5951=VERTEX_POINT('',#23990);
#5952=VERTEX_POINT('',#23992);
#5953=VERTEX_POINT('',#24031);
#5954=VERTEX_POINT('',#24058);
#5955=VERTEX_POINT('',#24060);
#5956=VERTEX_POINT('',#24143);
#5957=VERTEX_POINT('',#24151);
#5958=VERTEX_POINT('',#24174);
#5959=VERTEX_POINT('',#24257);
#5960=VERTEX_POINT('',#24350);
#5961=VERTEX_POINT('',#24423);
#5962=VERTEX_POINT('',#24430);
#5963=VERTEX_POINT('',#24431);
#5964=VERTEX_POINT('',#24433);
#5965=VERTEX_POINT('',#24435);
#5966=VERTEX_POINT('',#24478);
#5967=VERTEX_POINT('',#24483);
#5968=VERTEX_POINT('',#24514);
#5969=VERTEX_POINT('',#24516);
#5970=VERTEX_POINT('',#24518);
#5971=VERTEX_POINT('',#24520);
#5972=VERTEX_POINT('',#24533);
#5973=VERTEX_POINT('',#24540);
#5974=VERTEX_POINT('',#24549);
#5975=VERTEX_POINT('',#24558);
#7357=EDGE_CURVE('',#5896,#5897,#192,.T.);
#7358=EDGE_CURVE('',#5898,#5897,#193,.T.);
#7359=EDGE_CURVE('',#5898,#5899,#194,.T.);
#7360=EDGE_CURVE('',#5899,#5896,#3267,.T.);
#7361=EDGE_CURVE('',#5900,#5901,#195,.T.);
#7362=EDGE_CURVE('',#5902,#5901,#196,.T.);
#7363=EDGE_CURVE('',#5902,#5903,#197,.T.);
#7364=EDGE_CURVE('',#5903,#5900,#3268,.T.);
#7365=EDGE_CURVE('',#5901,#5904,#198,.T.);
#7366=EDGE_CURVE('',#5904,#5905,#3269,.T.);
#7367=EDGE_CURVE('',#5905,#5902,#199,.T.);
#7368=EDGE_CURVE('',#5906,#5907,#3270,.T.);
#7369=EDGE_CURVE('',#5907,#5908,#939,.T.);
#7370=EDGE_CURVE('',#5908,#5909,#3271,.T.);
#7371=EDGE_CURVE('',#5909,#5906,#940,.T.);
#7372=EDGE_CURVE('',#5908,#5905,#200,.T.);
#7373=EDGE_CURVE('',#5904,#5909,#201,.T.);
#7374=EDGE_CURVE('',#5897,#5910,#202,.T.);
#7375=EDGE_CURVE('',#5910,#5911,#3272,.T.);
#7376=EDGE_CURVE('',#5911,#5898,#203,.T.);
#7377=EDGE_CURVE('',#5910,#5907,#204,.T.);
#7378=EDGE_CURVE('',#5906,#5911,#205,.T.);
#7379=EDGE_CURVE('',#5896,#5912,#3273,.T.);
#7380=EDGE_CURVE('',#5912,#5913,#206,.T.);
#7381=EDGE_CURVE('',#5913,#5910,#3274,.T.);
#7382=EDGE_CURVE('',#5899,#5914,#3275,.T.);
#7383=EDGE_CURVE('',#5915,#5914,#3276,.T.);
#7384=EDGE_CURVE('',#5916,#5915,#3277,.T.);
#7385=EDGE_CURVE('',#5912,#5916,#3278,.T.);
#7386=EDGE_CURVE('',#5900,#5917,#3279,.T.);
#7387=EDGE_CURVE('',#5918,#5917,#207,.T.);
#7388=EDGE_CURVE('',#5919,#5918,#208,.T.);
#7389=EDGE_CURVE('',#5920,#5919,#209,.T.);
#7390=EDGE_CURVE('',#5921,#5920,#941,.T.);
#7391=EDGE_CURVE('',#5922,#5921,#210,.T.);
#7392=EDGE_CURVE('',#5923,#5922,#211,.T.);
#7393=EDGE_CURVE('',#5914,#5923,#212,.T.);
#7394=EDGE_CURVE('',#5924,#5925,#213,.T.);
#7395=EDGE_CURVE('',#5926,#5925,#214,.T.);
#7396=EDGE_CURVE('',#5926,#5927,#215,.T.);
#7397=EDGE_CURVE('',#5927,#5924,#3280,.T.);
#7398=EDGE_CURVE('',#5928,#5929,#216,.T.);
#7399=EDGE_CURVE('',#5930,#5929,#217,.T.);
#7400=EDGE_CURVE('',#5930,#5931,#218,.T.);
#7401=EDGE_CURVE('',#5931,#5928,#3281,.T.);
#7402=EDGE_CURVE('',#5929,#5932,#219,.T.);
#7403=EDGE_CURVE('',#5932,#5933,#3282,.T.);
#7404=EDGE_CURVE('',#5933,#5930,#220,.T.);
#7405=EDGE_CURVE('',#5934,#5935,#3283,.T.);
#7406=EDGE_CURVE('',#5935,#5936,#942,.T.);
#7407=EDGE_CURVE('',#5936,#5937,#3284,.T.);
#7408=EDGE_CURVE('',#5937,#5934,#943,.T.);
#7409=EDGE_CURVE('',#5936,#5933,#221,.T.);
#7410=EDGE_CURVE('',#5932,#5937,#222,.T.);
#7411=EDGE_CURVE('',#5925,#5938,#223,.T.);
#7412=EDGE_CURVE('',#5938,#5939,#3285,.T.);
#7413=EDGE_CURVE('',#5939,#5926,#224,.T.);
#7414=EDGE_CURVE('',#5938,#5935,#225,.T.);
#7415=EDGE_CURVE('',#5934,#5939,#226,.T.);
#7416=EDGE_CURVE('',#5940,#5931,#3286,.T.);
#7417=EDGE_CURVE('',#5940,#5941,#3287,.T.);
#7418=EDGE_CURVE('',#5942,#5941,#3288,.T.);
#7419=EDGE_CURVE('',#5943,#5942,#3289,.T.);
#7420=EDGE_CURVE('',#5928,#5943,#3290,.T.);
#7421=EDGE_CURVE('',#5933,#5944,#3291,.T.);
#7422=EDGE_CURVE('',#5944,#5940,#227,.T.);
#7423=EDGE_CURVE('',#5913,#5945,#944,.T.);
#7424=EDGE_CURVE('',#5946,#5945,#3292,.T.);
#7425=EDGE_CURVE('',#5946,#5944,#945,.T.);
#7426=EDGE_CURVE('',#5905,#5938,#3293,.T.);
#7427=EDGE_CURVE('',#5947,#5948,#228,.T.);
#7428=EDGE_CURVE('',#5918,#5948,#229,.T.);
#7429=EDGE_CURVE('',#5917,#5947,#3294,.T.);
#7430=EDGE_CURVE('',#5949,#5923,#230,.T.);
#7431=EDGE_CURVE('',#5949,#5915,#231,.T.);
#7432=EDGE_CURVE('',#5922,#5950,#3295,.T.);
#7433=EDGE_CURVE('',#5950,#5949,#232,.T.);
#7434=EDGE_CURVE('',#5920,#5951,#3296,.T.);
#7435=EDGE_CURVE('',#5951,#5952,#946,.T.);
#7436=EDGE_CURVE('',#5952,#5921,#3297,.T.);
#7437=EDGE_CURVE('',#5952,#5950,#233,.T.);
#7438=EDGE_CURVE('',#5948,#5953,#234,.T.);
#7439=EDGE_CURVE('',#5953,#5919,#3298,.T.);
#7440=EDGE_CURVE('',#5953,#5951,#235,.T.);
#7441=EDGE_CURVE('',#5947,#5954,#3299,.T.);
#7442=EDGE_CURVE('',#5955,#5954,#236,.T.);
#7443=EDGE_CURVE('',#5956,#5955,#237,.T.);
#7444=EDGE_CURVE('',#5956,#5953,#3300,.T.);
#7445=EDGE_CURVE('',#5924,#5903,#3301,.T.);
#7446=EDGE_CURVE('',#5927,#5957,#3302,.T.);
#7447=EDGE_CURVE('',#5954,#5957,#3303,.T.);
#7448=EDGE_CURVE('',#5942,#5958,#238,.T.);
#7449=EDGE_CURVE('',#5959,#5958,#239,.T.);
#7450=EDGE_CURVE('',#5959,#5943,#240,.T.);
#7451=EDGE_CURVE('',#5957,#5960,#241,.T.);
#7452=EDGE_CURVE('',#5955,#5960,#242,.T.);
#7453=EDGE_CURVE('',#5960,#5961,#243,.T.);
#7454=EDGE_CURVE('',#5961,#5956,#3304,.T.);
#7455=EDGE_CURVE('',#5962,#5963,#3305,.T.);
#7456=EDGE_CURVE('',#5963,#5964,#947,.T.);
#7457=EDGE_CURVE('',#5964,#5965,#3306,.T.);
#7458=EDGE_CURVE('',#5965,#5962,#948,.T.);
#7459=EDGE_CURVE('',#5964,#5956,#244,.T.);
#7460=EDGE_CURVE('',#5961,#5965,#245,.T.);
#7461=EDGE_CURVE('',#5958,#5966,#246,.T.);
#7462=EDGE_CURVE('',#5966,#5967,#3307,.T.);
#7463=EDGE_CURVE('',#5967,#5959,#247,.T.);
#7464=EDGE_CURVE('',#5966,#5963,#248,.T.);
#7465=EDGE_CURVE('',#5962,#5967,#249,.T.);
#7466=EDGE_CURVE('',#5968,#5966,#3308,.T.);
#7467=EDGE_CURVE('',#5968,#5969,#949,.T.);
#7468=EDGE_CURVE('',#5970,#5969,#3309,.T.);
#7469=EDGE_CURVE('',#5970,#5971,#950,.T.);
#7470=EDGE_CURVE('',#5950,#5971,#3310,.T.);
#7471=EDGE_CURVE('',#5941,#5968,#250,.T.);
#7472=EDGE_CURVE('',#5972,#5946,#251,.T.);
#7473=EDGE_CURVE('',#5972,#5973,#3311,.T.);
#7474=EDGE_CURVE('',#5969,#5973,#252,.T.);
#7475=EDGE_CURVE('',#5974,#5970,#253,.T.);
#7476=EDGE_CURVE('',#5973,#5974,#3312,.T.);
#7477=EDGE_CURVE('',#5975,#5974,#3313,.T.);
#7478=EDGE_CURVE('',#5945,#5975,#254,.T.);
#7479=EDGE_CURVE('',#5971,#5916,#255,.T.);
#7480=EDGE_CURVE('',#5975,#5972,#3314,.T.);
#9961=ORIENTED_EDGE('',*,*,#7357,.T.);
#9962=ORIENTED_EDGE('',*,*,#7358,.F.);
#9963=ORIENTED_EDGE('',*,*,#7359,.T.);
#9964=ORIENTED_EDGE('',*,*,#7360,.T.);
#9965=ORIENTED_EDGE('',*,*,#7361,.T.);
#9966=ORIENTED_EDGE('',*,*,#7362,.F.);
#9967=ORIENTED_EDGE('',*,*,#7363,.T.);
#9968=ORIENTED_EDGE('',*,*,#7364,.T.);
#9969=ORIENTED_EDGE('',*,*,#7362,.T.);
#9970=ORIENTED_EDGE('',*,*,#7365,.T.);
#9971=ORIENTED_EDGE('',*,*,#7366,.T.);
#9972=ORIENTED_EDGE('',*,*,#7367,.T.);
#9973=ORIENTED_EDGE('',*,*,#7368,.T.);
#9974=ORIENTED_EDGE('',*,*,#7369,.T.);
#9975=ORIENTED_EDGE('',*,*,#7370,.T.);
#9976=ORIENTED_EDGE('',*,*,#7371,.T.);
#9977=ORIENTED_EDGE('',*,*,#7370,.F.);
#9978=ORIENTED_EDGE('',*,*,#7372,.T.);
#9979=ORIENTED_EDGE('',*,*,#7366,.F.);
#9980=ORIENTED_EDGE('',*,*,#7373,.T.);
#9981=ORIENTED_EDGE('',*,*,#7358,.T.);
#9982=ORIENTED_EDGE('',*,*,#7374,.T.);
#9983=ORIENTED_EDGE('',*,*,#7375,.T.);
#9984=ORIENTED_EDGE('',*,*,#7376,.T.);
#9985=ORIENTED_EDGE('',*,*,#7375,.F.);
#9986=ORIENTED_EDGE('',*,*,#7377,.T.);
#9987=ORIENTED_EDGE('',*,*,#7368,.F.);
#9988=ORIENTED_EDGE('',*,*,#7378,.T.);
#9989=ORIENTED_EDGE('',*,*,#7374,.F.);
#9990=ORIENTED_EDGE('',*,*,#7357,.F.);
#9991=ORIENTED_EDGE('',*,*,#7379,.T.);
#9992=ORIENTED_EDGE('',*,*,#7380,.T.);
#9993=ORIENTED_EDGE('',*,*,#7381,.T.);
#9994=ORIENTED_EDGE('',*,*,#7360,.F.);
#9995=ORIENTED_EDGE('',*,*,#7382,.T.);
#9996=ORIENTED_EDGE('',*,*,#7383,.F.);
#9997=ORIENTED_EDGE('',*,*,#7384,.F.);
#9998=ORIENTED_EDGE('',*,*,#7385,.F.);
#9999=ORIENTED_EDGE('',*,*,#7379,.F.);
#10000=ORIENTED_EDGE('',*,*,#7359,.F.);
#10001=ORIENTED_EDGE('',*,*,#7376,.F.);
#10002=ORIENTED_EDGE('',*,*,#7378,.F.);
#10003=ORIENTED_EDGE('',*,*,#7371,.F.);
#10004=ORIENTED_EDGE('',*,*,#7373,.F.);
#10005=ORIENTED_EDGE('',*,*,#7365,.F.);
#10006=ORIENTED_EDGE('',*,*,#7361,.F.);
#10007=ORIENTED_EDGE('',*,*,#7386,.T.);
#10008=ORIENTED_EDGE('',*,*,#7387,.F.);
#10009=ORIENTED_EDGE('',*,*,#7388,.F.);
#10010=ORIENTED_EDGE('',*,*,#7389,.F.);
#10011=ORIENTED_EDGE('',*,*,#7390,.F.);
#10012=ORIENTED_EDGE('',*,*,#7391,.F.);
#10013=ORIENTED_EDGE('',*,*,#7392,.F.);
#10014=ORIENTED_EDGE('',*,*,#7393,.F.);
#10015=ORIENTED_EDGE('',*,*,#7382,.F.);
#10016=ORIENTED_EDGE('',*,*,#7394,.T.);
#10017=ORIENTED_EDGE('',*,*,#7395,.F.);
#10018=ORIENTED_EDGE('',*,*,#7396,.T.);
#10019=ORIENTED_EDGE('',*,*,#7397,.T.);
#10020=ORIENTED_EDGE('',*,*,#7398,.T.);
#10021=ORIENTED_EDGE('',*,*,#7399,.F.);
#10022=ORIENTED_EDGE('',*,*,#7400,.T.);
#10023=ORIENTED_EDGE('',*,*,#7401,.T.);
#10024=ORIENTED_EDGE('',*,*,#7399,.T.);
#10025=ORIENTED_EDGE('',*,*,#7402,.T.);
#10026=ORIENTED_EDGE('',*,*,#7403,.T.);
#10027=ORIENTED_EDGE('',*,*,#7404,.T.);
#10028=ORIENTED_EDGE('',*,*,#7405,.T.);
#10029=ORIENTED_EDGE('',*,*,#7406,.T.);
#10030=ORIENTED_EDGE('',*,*,#7407,.T.);
#10031=ORIENTED_EDGE('',*,*,#7408,.T.);
#10032=ORIENTED_EDGE('',*,*,#7407,.F.);
#10033=ORIENTED_EDGE('',*,*,#7409,.T.);
#10034=ORIENTED_EDGE('',*,*,#7403,.F.);
#10035=ORIENTED_EDGE('',*,*,#7410,.T.);
#10036=ORIENTED_EDGE('',*,*,#7395,.T.);
#10037=ORIENTED_EDGE('',*,*,#7411,.T.);
#10038=ORIENTED_EDGE('',*,*,#7412,.T.);
#10039=ORIENTED_EDGE('',*,*,#7413,.T.);
#10040=ORIENTED_EDGE('',*,*,#7412,.F.);
#10041=ORIENTED_EDGE('',*,*,#7414,.T.);
#10042=ORIENTED_EDGE('',*,*,#7405,.F.);
#10043=ORIENTED_EDGE('',*,*,#7415,.T.);
#10044=ORIENTED_EDGE('',*,*,#7401,.F.);
#10045=ORIENTED_EDGE('',*,*,#7416,.F.);
#10046=ORIENTED_EDGE('',*,*,#7417,.T.);
#10047=ORIENTED_EDGE('',*,*,#7418,.F.);
#10048=ORIENTED_EDGE('',*,*,#7419,.F.);
#10049=ORIENTED_EDGE('',*,*,#7420,.F.);
#10050=ORIENTED_EDGE('',*,*,#7400,.F.);
#10051=ORIENTED_EDGE('',*,*,#7404,.F.);
#10052=ORIENTED_EDGE('',*,*,#7421,.T.);
#10053=ORIENTED_EDGE('',*,*,#7422,.T.);
#10054=ORIENTED_EDGE('',*,*,#7416,.T.);
#10055=ORIENTED_EDGE('',*,*,#7377,.F.);
#10056=ORIENTED_EDGE('',*,*,#7381,.F.);
#10057=ORIENTED_EDGE('',*,*,#7423,.T.);
#10058=ORIENTED_EDGE('',*,*,#7424,.F.);
#10059=ORIENTED_EDGE('',*,*,#7425,.T.);
#10060=ORIENTED_EDGE('',*,*,#7421,.F.);
#10061=ORIENTED_EDGE('',*,*,#7409,.F.);
#10062=ORIENTED_EDGE('',*,*,#7406,.F.);
#10063=ORIENTED_EDGE('',*,*,#7414,.F.);
#10064=ORIENTED_EDGE('',*,*,#7426,.F.);
#10065=ORIENTED_EDGE('',*,*,#7372,.F.);
#10066=ORIENTED_EDGE('',*,*,#7369,.F.);
#10067=ORIENTED_EDGE('',*,*,#7427,.T.);
#10068=ORIENTED_EDGE('',*,*,#7428,.F.);
#10069=ORIENTED_EDGE('',*,*,#7387,.T.);
#10070=ORIENTED_EDGE('',*,*,#7429,.T.);
#10071=ORIENTED_EDGE('',*,*,#7393,.T.);
#10072=ORIENTED_EDGE('',*,*,#7430,.F.);
#10073=ORIENTED_EDGE('',*,*,#7431,.T.);
#10074=ORIENTED_EDGE('',*,*,#7383,.T.);
#10075=ORIENTED_EDGE('',*,*,#7430,.T.);
#10076=ORIENTED_EDGE('',*,*,#7392,.T.);
#10077=ORIENTED_EDGE('',*,*,#7432,.T.);
#10078=ORIENTED_EDGE('',*,*,#7433,.T.);
#10079=ORIENTED_EDGE('',*,*,#7434,.T.);
#10080=ORIENTED_EDGE('',*,*,#7435,.T.);
#10081=ORIENTED_EDGE('',*,*,#7436,.T.);
#10082=ORIENTED_EDGE('',*,*,#7390,.T.);
#10083=ORIENTED_EDGE('',*,*,#7436,.F.);
#10084=ORIENTED_EDGE('',*,*,#7437,.T.);
#10085=ORIENTED_EDGE('',*,*,#7432,.F.);
#10086=ORIENTED_EDGE('',*,*,#7391,.T.);
#10087=ORIENTED_EDGE('',*,*,#7428,.T.);
#10088=ORIENTED_EDGE('',*,*,#7438,.T.);
#10089=ORIENTED_EDGE('',*,*,#7439,.T.);
#10090=ORIENTED_EDGE('',*,*,#7388,.T.);
#10091=ORIENTED_EDGE('',*,*,#7439,.F.);
#10092=ORIENTED_EDGE('',*,*,#7440,.T.);
#10093=ORIENTED_EDGE('',*,*,#7434,.F.);
#10094=ORIENTED_EDGE('',*,*,#7389,.T.);
#10095=ORIENTED_EDGE('',*,*,#7438,.F.);
#10096=ORIENTED_EDGE('',*,*,#7427,.F.);
#10097=ORIENTED_EDGE('',*,*,#7441,.T.);
#10098=ORIENTED_EDGE('',*,*,#7442,.F.);
#10099=ORIENTED_EDGE('',*,*,#7443,.F.);
#10100=ORIENTED_EDGE('',*,*,#7444,.T.);
#10101=ORIENTED_EDGE('',*,*,#7364,.F.);
#10102=ORIENTED_EDGE('',*,*,#7445,.F.);
#10103=ORIENTED_EDGE('',*,*,#7397,.F.);
#10104=ORIENTED_EDGE('',*,*,#7446,.T.);
#10105=ORIENTED_EDGE('',*,*,#7447,.F.);
#10106=ORIENTED_EDGE('',*,*,#7441,.F.);
#10107=ORIENTED_EDGE('',*,*,#7429,.F.);
#10108=ORIENTED_EDGE('',*,*,#7386,.F.);
#10109=ORIENTED_EDGE('',*,*,#7448,.T.);
#10110=ORIENTED_EDGE('',*,*,#7449,.F.);
#10111=ORIENTED_EDGE('',*,*,#7450,.T.);
#10112=ORIENTED_EDGE('',*,*,#7419,.T.);
#10113=ORIENTED_EDGE('',*,*,#7451,.T.);
#10114=ORIENTED_EDGE('',*,*,#7452,.F.);
#10115=ORIENTED_EDGE('',*,*,#7442,.T.);
#10116=ORIENTED_EDGE('',*,*,#7447,.T.);
#10117=ORIENTED_EDGE('',*,*,#7452,.T.);
#10118=ORIENTED_EDGE('',*,*,#7453,.T.);
#10119=ORIENTED_EDGE('',*,*,#7454,.T.);
#10120=ORIENTED_EDGE('',*,*,#7443,.T.);
#10121=ORIENTED_EDGE('',*,*,#7455,.T.);
#10122=ORIENTED_EDGE('',*,*,#7456,.T.);
#10123=ORIENTED_EDGE('',*,*,#7457,.T.);
#10124=ORIENTED_EDGE('',*,*,#7458,.T.);
#10125=ORIENTED_EDGE('',*,*,#7457,.F.);
#10126=ORIENTED_EDGE('',*,*,#7459,.T.);
#10127=ORIENTED_EDGE('',*,*,#7454,.F.);
#10128=ORIENTED_EDGE('',*,*,#7460,.T.);
#10129=ORIENTED_EDGE('',*,*,#7449,.T.);
#10130=ORIENTED_EDGE('',*,*,#7461,.T.);
#10131=ORIENTED_EDGE('',*,*,#7462,.T.);
#10132=ORIENTED_EDGE('',*,*,#7463,.T.);
#10133=ORIENTED_EDGE('',*,*,#7462,.F.);
#10134=ORIENTED_EDGE('',*,*,#7464,.T.);
#10135=ORIENTED_EDGE('',*,*,#7455,.F.);
#10136=ORIENTED_EDGE('',*,*,#7465,.T.);
#10137=ORIENTED_EDGE('',*,*,#7440,.F.);
#10138=ORIENTED_EDGE('',*,*,#7444,.F.);
#10139=ORIENTED_EDGE('',*,*,#7459,.F.);
#10140=ORIENTED_EDGE('',*,*,#7456,.F.);
#10141=ORIENTED_EDGE('',*,*,#7464,.F.);
#10142=ORIENTED_EDGE('',*,*,#7466,.F.);
#10143=ORIENTED_EDGE('',*,*,#7467,.T.);
#10144=ORIENTED_EDGE('',*,*,#7468,.F.);
#10145=ORIENTED_EDGE('',*,*,#7469,.T.);
#10146=ORIENTED_EDGE('',*,*,#7470,.F.);
#10147=ORIENTED_EDGE('',*,*,#7437,.F.);
#10148=ORIENTED_EDGE('',*,*,#7435,.F.);
#10149=ORIENTED_EDGE('',*,*,#7398,.F.);
#10150=ORIENTED_EDGE('',*,*,#7420,.T.);
#10151=ORIENTED_EDGE('',*,*,#7450,.F.);
#10152=ORIENTED_EDGE('',*,*,#7463,.F.);
#10153=ORIENTED_EDGE('',*,*,#7465,.F.);
#10154=ORIENTED_EDGE('',*,*,#7458,.F.);
#10155=ORIENTED_EDGE('',*,*,#7460,.F.);
#10156=ORIENTED_EDGE('',*,*,#7453,.F.);
#10157=ORIENTED_EDGE('',*,*,#7451,.F.);
#10158=ORIENTED_EDGE('',*,*,#7446,.F.);
#10159=ORIENTED_EDGE('',*,*,#7396,.F.);
#10160=ORIENTED_EDGE('',*,*,#7413,.F.);
#10161=ORIENTED_EDGE('',*,*,#7415,.F.);
#10162=ORIENTED_EDGE('',*,*,#7408,.F.);
#10163=ORIENTED_EDGE('',*,*,#7410,.F.);
#10164=ORIENTED_EDGE('',*,*,#7402,.F.);
#10165=ORIENTED_EDGE('',*,*,#7367,.F.);
#10166=ORIENTED_EDGE('',*,*,#7426,.T.);
#10167=ORIENTED_EDGE('',*,*,#7411,.F.);
#10168=ORIENTED_EDGE('',*,*,#7394,.F.);
#10169=ORIENTED_EDGE('',*,*,#7445,.T.);
#10170=ORIENTED_EDGE('',*,*,#7363,.F.);
#10171=ORIENTED_EDGE('',*,*,#7448,.F.);
#10172=ORIENTED_EDGE('',*,*,#7418,.T.);
#10173=ORIENTED_EDGE('',*,*,#7471,.T.);
#10174=ORIENTED_EDGE('',*,*,#7466,.T.);
#10175=ORIENTED_EDGE('',*,*,#7461,.F.);
#10176=ORIENTED_EDGE('',*,*,#7471,.F.);
#10177=ORIENTED_EDGE('',*,*,#7417,.F.);
#10178=ORIENTED_EDGE('',*,*,#7422,.F.);
#10179=ORIENTED_EDGE('',*,*,#7425,.F.);
#10180=ORIENTED_EDGE('',*,*,#7472,.F.);
#10181=ORIENTED_EDGE('',*,*,#7473,.T.);
#10182=ORIENTED_EDGE('',*,*,#7474,.F.);
#10183=ORIENTED_EDGE('',*,*,#7467,.F.);
#10184=ORIENTED_EDGE('',*,*,#7475,.T.);
#10185=ORIENTED_EDGE('',*,*,#7468,.T.);
#10186=ORIENTED_EDGE('',*,*,#7474,.T.);
#10187=ORIENTED_EDGE('',*,*,#7476,.T.);
#10188=ORIENTED_EDGE('',*,*,#7475,.F.);
#10189=ORIENTED_EDGE('',*,*,#7477,.F.);
#10190=ORIENTED_EDGE('',*,*,#7478,.F.);
#10191=ORIENTED_EDGE('',*,*,#7423,.F.);
#10192=ORIENTED_EDGE('',*,*,#7380,.F.);
#10193=ORIENTED_EDGE('',*,*,#7385,.T.);
#10194=ORIENTED_EDGE('',*,*,#7479,.F.);
#10195=ORIENTED_EDGE('',*,*,#7469,.F.);
#10196=ORIENTED_EDGE('',*,*,#7476,.F.);
#10197=ORIENTED_EDGE('',*,*,#7473,.F.);
#10198=ORIENTED_EDGE('',*,*,#7480,.F.);
#10199=ORIENTED_EDGE('',*,*,#7477,.T.);
#10200=ORIENTED_EDGE('',*,*,#7472,.T.);
#10201=ORIENTED_EDGE('',*,*,#7424,.T.);
#10202=ORIENTED_EDGE('',*,*,#7478,.T.);
#10203=ORIENTED_EDGE('',*,*,#7480,.T.);
#10204=ORIENTED_EDGE('',*,*,#7433,.F.);
#10205=ORIENTED_EDGE('',*,*,#7470,.T.);
#10206=ORIENTED_EDGE('',*,*,#7479,.T.);
#10207=ORIENTED_EDGE('',*,*,#7384,.T.);
#10208=ORIENTED_EDGE('',*,*,#7431,.F.);
#12699=PLANE('',#14383);
#12700=PLANE('',#14389);
#12701=PLANE('',#14391);
#12702=PLANE('',#14397);
#12703=PLANE('',#14401);
#12704=PLANE('',#14410);
#13278=ADVANCED_FACE('',(#1515),#447,.T.);
#13279=ADVANCED_FACE('',(#1516),#448,.T.);
#13280=ADVANCED_FACE('',(#1517),#449,.T.);
#13281=ADVANCED_FACE('',(#1518),#1177,.T.);
#13282=ADVANCED_FACE('',(#1519),#450,.T.);
#13283=ADVANCED_FACE('',(#1520),#451,.T.);
#13284=ADVANCED_FACE('',(#1521),#452,.T.);
#13285=ADVANCED_FACE('',(#1522),#706,.T.);
#13286=ADVANCED_FACE('',(#1523),#12699,.T.);
#13287=ADVANCED_FACE('',(#1524),#707,.T.);
#13288=ADVANCED_FACE('',(#1525),#453,.T.);
#13289=ADVANCED_FACE('',(#1526),#454,.T.);
#13290=ADVANCED_FACE('',(#1527),#455,.T.);
#13291=ADVANCED_FACE('',(#1528),#1178,.T.);
#13292=ADVANCED_FACE('',(#1529),#456,.T.);
#13293=ADVANCED_FACE('',(#1530),#457,.T.);
#13294=ADVANCED_FACE('',(#1531),#458,.T.);
#13295=ADVANCED_FACE('',(#1532),#12700,.T.);
#13296=ADVANCED_FACE('',(#1533),#708,.T.);
#13297=ADVANCED_FACE('',(#1534),#12701,.T.);
#13298=ADVANCED_FACE('',(#1535),#459,.T.);
#13299=ADVANCED_FACE('',(#1536),#460,.T.);
#13300=ADVANCED_FACE('',(#1537),#461,.T.);
#13301=ADVANCED_FACE('',(#1538),#1179,.T.);
#13302=ADVANCED_FACE('',(#1539),#462,.T.);
#13303=ADVANCED_FACE('',(#1540),#463,.T.);
#13304=ADVANCED_FACE('',(#1541),#464,.T.);
#13305=ADVANCED_FACE('',(#1542),#709,.T.);
#13306=ADVANCED_FACE('',(#1543),#12702,.T.);
#13307=ADVANCED_FACE('',(#1544),#465,.T.);
#13308=ADVANCED_FACE('',(#1545),#466,.T.);
#13309=ADVANCED_FACE('',(#1546),#467,.T.);
#13310=ADVANCED_FACE('',(#1547),#1180,.T.);
#13311=ADVANCED_FACE('',(#1548),#468,.T.);
#13312=ADVANCED_FACE('',(#1549),#469,.T.);
#13313=ADVANCED_FACE('',(#1550),#470,.T.);
#13314=ADVANCED_FACE('',(#1551),#12703,.F.);
#13315=ADVANCED_FACE('',(#1552),#710,.T.);
#13316=ADVANCED_FACE('',(#1553),#711,.T.);
#13317=ADVANCED_FACE('',(#1554),#712,.T.);
#13318=ADVANCED_FACE('',(#1555),#713,.T.);
#13319=ADVANCED_FACE('',(#1556),#714,.T.);
#13320=ADVANCED_FACE('',(#1557),#715,.T.);
#13321=ADVANCED_FACE('',(#1558),#12704,.T.);
#13322=ADVANCED_FACE('',(#1559),#716,.T.);
#13323=ADVANCED_FACE('',(#1560),#717,.T.);
#13809=CLOSED_SHELL('',(#13278,#13279,#13280,#13281,#13282,#13283,#13284,
#13285,#13286,#13287,#13288,#13289,#13290,#13291,#13292,#13293,#13294,#13295,
#13296,#13297,#13298,#13299,#13300,#13301,#13302,#13303,#13304,#13305,#13306,
#13307,#13308,#13309,#13310,#13311,#13312,#13313,#13314,#13315,#13316,#13317,
#13318,#13319,#13320,#13321,#13322,#13323));
#14378=AXIS2_PLACEMENT_3D('',#22641,#16185,#16186);
#14379=AXIS2_PLACEMENT_3D('',#23011,#16190,#16191);
#14380=AXIS2_PLACEMENT_3D('',#23016,#16193,#16194);
#14381=AXIS2_PLACEMENT_3D('',#23019,#16196,#16197);
#14382=AXIS2_PLACEMENT_3D('',#23107,#16199,#16200);
#14383=AXIS2_PLACEMENT_3D('',#23118,#16203,#16204);
#14384=AXIS2_PLACEMENT_3D('',#23126,#16209,#16210);
#14385=AXIS2_PLACEMENT_3D('',#23193,#16212,#16213);
#14386=AXIS2_PLACEMENT_3D('',#23625,#16217,#16218);
#14387=AXIS2_PLACEMENT_3D('',#23630,#16220,#16221);
#14388=AXIS2_PLACEMENT_3D('',#23633,#16223,#16224);
#14389=AXIS2_PLACEMENT_3D('',#23709,#16226,#16227);
#14390=AXIS2_PLACEMENT_3D('',#23719,#16233,#16234);
#14391=AXIS2_PLACEMENT_3D('',#23728,#16236,#16237);
#14392=AXIS2_PLACEMENT_3D('',#23730,#16238,#16239);
#14393=AXIS2_PLACEMENT_3D('',#23733,#16241,#16242);
#14394=AXIS2_PLACEMENT_3D('',#23989,#16246,#16247);
#14395=AXIS2_PLACEMENT_3D('',#23993,#16249,#16250);
#14396=AXIS2_PLACEMENT_3D('',#24057,#16253,#16254);
#14397=AXIS2_PLACEMENT_3D('',#24149,#16257,#16258);
#14398=AXIS2_PLACEMENT_3D('',#24429,#16263,#16264);
#14399=AXIS2_PLACEMENT_3D('',#24434,#16266,#16267);
#14400=AXIS2_PLACEMENT_3D('',#24437,#16269,#16270);
#14401=AXIS2_PLACEMENT_3D('',#24513,#16272,#16273);
#14402=AXIS2_PLACEMENT_3D('',#24517,#16275,#16276);
#14403=AXIS2_PLACEMENT_3D('',#24521,#16278,#16279);
#14404=AXIS2_PLACEMENT_3D('',#24523,#16281,#16282);
#14405=AXIS2_PLACEMENT_3D('',#24524,#16283,#16284);
#14406=AXIS2_PLACEMENT_3D('',#24525,#16285,#16286);
#14407=AXIS2_PLACEMENT_3D('',#24532,#16287,#16288);
#14408=AXIS2_PLACEMENT_3D('',#24548,#16290,#16291);
#14409=AXIS2_PLACEMENT_3D('',#24557,#16293,#16294);
#14410=AXIS2_PLACEMENT_3D('',#24572,#16296,#16297);
#14411=AXIS2_PLACEMENT_3D('',#24574,#16299,#16300);
#14412=AXIS2_PLACEMENT_3D('',#24575,#16301,#16302);
#16185=DIRECTION('axis',(0.,0.,1.));
#16186=DIRECTION('refdir',(1.,0.,0.));
#16187=DIRECTION('',(0.342997170285005,0.939336436627729,0.));
#16188=DIRECTION('',(-0.342997170285022,-6.70692126230321E-16,-0.939336436627723));
#16189=DIRECTION('',(0.737980838656825,0.568079932640029,0.364238207643117));
#16190=DIRECTION('center_axis',(-1.,0.,0.));
#16191=DIRECTION('ref_axis',(0.,-1.,0.));
#16192=DIRECTION('',(0.707106781186544,0.352766841475276,0.612825877028347));
#16193=DIRECTION('center_axis',(-1.,0.,0.));
#16194=DIRECTION('ref_axis',(0.,-1.,0.));
#16195=DIRECTION('',(-0.707106781186552,-0.612825877028345,-0.352766841475263));
#16196=DIRECTION('center_axis',(1.,0.,0.));
#16197=DIRECTION('ref_axis',(0.,-1.,0.));
#16198=DIRECTION('',(-0.737980838656826,-0.364238207643135,-0.568079932640015));
#16199=DIRECTION('center_axis',(0.,1.,0.));
#16200=DIRECTION('ref_axis',(0.70710678118654,0.,-0.707106781186555));
#16201=DIRECTION('',(0.,1.,0.));
#16202=DIRECTION('',(0.,-1.,0.));
#16203=DIRECTION('center_axis',(0.,0.,-1.));
#16204=DIRECTION('ref_axis',(0.,-1.,0.));
#16205=DIRECTION('',(-1.,0.,0.));
#16206=DIRECTION('',(0.342997170284996,-0.939336436627732,0.));
#16207=DIRECTION('',(0.,-1.,0.));
#16208=DIRECTION('',(-1.,0.,0.));
#16209=DIRECTION('center_axis',(-1.,0.,0.));
#16210=DIRECTION('ref_axis',(0.,-1.,0.));
#16211=DIRECTION('',(-1.,0.,0.));
#16212=DIRECTION('center_axis',(-1.,0.,0.));
#16213=DIRECTION('ref_axis',(0.,-1.,0.));
#16214=DIRECTION('',(0.342997170285042,-2.68276850492132E-15,-0.939336436627715));
#16215=DIRECTION('',(-0.342997170285017,-0.939336436627724,0.));
#16216=DIRECTION('',(0.737980838656834,0.364238207643121,-0.568079932640014));
#16217=DIRECTION('center_axis',(-1.,0.,0.));
#16218=DIRECTION('ref_axis',(0.,-1.29526019539602E-15,1.));
#16219=DIRECTION('',(0.707106781186544,0.612825877028338,-0.352766841475291));
#16220=DIRECTION('center_axis',(-1.,0.,0.));
#16221=DIRECTION('ref_axis',(0.,-1.29526019539601E-15,1.));
#16222=DIRECTION('',(-0.707106781186543,-0.352766841475279,0.612825877028346));
#16223=DIRECTION('center_axis',(1.,0.,0.));
#16224=DIRECTION('ref_axis',(0.,-1.29526019539602E-15,1.));
#16225=DIRECTION('',(-0.737980838656842,-0.568079932640019,0.364238207643096));
#16226=DIRECTION('center_axis',(0.,0.,1.));
#16227=DIRECTION('ref_axis',(0.,1.,0.));
#16228=DIRECTION('',(0.,-1.,0.));
#16229=DIRECTION('',(-1.,0.,0.));
#16230=DIRECTION('',(0.,1.,0.));
#16231=DIRECTION('',(-0.342997170285038,0.939336436627717,0.));
#16232=DIRECTION('',(-1.,0.,0.));
#16233=DIRECTION('center_axis',(0.,-1.,0.));
#16234=DIRECTION('ref_axis',(0.707106781186548,0.,0.707106781186548));
#16235=DIRECTION('',(0.,1.,0.));
#16236=DIRECTION('center_axis',(1.,0.,0.));
#16237=DIRECTION('ref_axis',(0.,0.,-1.));
#16238=DIRECTION('center_axis',(1.,0.,0.));
#16239=DIRECTION('ref_axis',(0.,-2.96059473233375E-15,-1.));
#16240=DIRECTION('',(0.,0.,-1.));
#16241=DIRECTION('center_axis',(1.,0.,0.));
#16242=DIRECTION('ref_axis',(0.,1.,-3.7007434154172E-15));
#16243=DIRECTION('',(0.,0.,1.));
#16244=DIRECTION('',(-0.342997170285022,6.70692126230321E-16,0.939336436627723));
#16245=DIRECTION('',(-0.737980838656832,0.364238207643115,0.56807993264002));
#16246=DIRECTION('center_axis',(1.,0.,0.));
#16247=DIRECTION('ref_axis',(0.,-1.,0.));
#16248=DIRECTION('',(-0.707106781186552,0.612825877028345,0.352766841475263));
#16249=DIRECTION('center_axis',(1.,0.,0.));
#16250=DIRECTION('ref_axis',(0.,-1.,0.));
#16251=DIRECTION('',(0.707106781186544,-0.352766841475276,-0.612825877028347));
#16252=DIRECTION('',(0.737980838656822,-0.568079932640023,-0.364238207643131));
#16253=DIRECTION('center_axis',(0.,0.,1.));
#16254=DIRECTION('ref_axis',(-0.707106781186548,-0.707106781186548,0.));
#16255=DIRECTION('',(0.,0.,1.));
#16256=DIRECTION('',(0.,0.,-1.));
#16257=DIRECTION('center_axis',(0.,-1.,0.));
#16258=DIRECTION('ref_axis',(0.,0.,1.));
#16259=DIRECTION('',(0.,0.,-1.));
#16260=DIRECTION('',(-1.,0.,0.));
#16261=DIRECTION('',(0.342997170285042,2.68276850492132E-15,0.939336436627715));
#16262=DIRECTION('',(-0.737980838656821,0.568079932640026,-0.36423820764313));
#16263=DIRECTION('center_axis',(1.,0.,0.));
#16264=DIRECTION('ref_axis',(0.,-1.29526019539602E-15,1.));
#16265=DIRECTION('',(-0.707106781186543,0.352766841475279,-0.612825877028346));
#16266=DIRECTION('center_axis',(1.,0.,0.));
#16267=DIRECTION('ref_axis',(0.,-1.29526019539601E-15,1.));
#16268=DIRECTION('',(0.707106781186544,-0.612825877028338,0.352766841475291));
#16269=DIRECTION('center_axis',(-1.,0.,0.));
#16270=DIRECTION('ref_axis',(0.,-1.29526019539602E-15,1.));
#16271=DIRECTION('',(0.737980838656848,-0.36423820764311,0.568079932640002));
#16272=DIRECTION('center_axis',(1.,0.,0.));
#16273=DIRECTION('ref_axis',(0.,0.,-1.));
#16274=DIRECTION('',(0.,-1.,0.));
#16275=DIRECTION('center_axis',(-1.,0.,0.));
#16276=DIRECTION('ref_axis',(0.,1.,-3.7007434154172E-15));
#16277=DIRECTION('',(0.,0.,1.));
#16278=DIRECTION('center_axis',(-1.,0.,0.));
#16279=DIRECTION('ref_axis',(0.,-2.96059473233375E-15,-1.));
#16280=DIRECTION('',(0.,1.,0.));
#16281=DIRECTION('center_axis',(-1.,0.,0.));
#16282=DIRECTION('ref_axis',(0.,-1.29526019539602E-15,1.));
#16283=DIRECTION('center_axis',(0.,0.,-1.));
#16284=DIRECTION('ref_axis',(0.707106781186548,-0.707106781186548,0.));
#16285=DIRECTION('center_axis',(0.,1.,0.));
#16286=DIRECTION('ref_axis',(-0.707106781186548,0.,0.707106781186548));
#16287=DIRECTION('center_axis',(-1.,0.,0.));
#16288=DIRECTION('ref_axis',(0.,1.,-3.7007434154172E-15));
#16289=DIRECTION('',(-1.,0.,0.));
#16290=DIRECTION('center_axis',(0.,0.,-1.));
#16291=DIRECTION('ref_axis',(-0.70710678118654,0.707106781186555,0.));
#16292=DIRECTION('',(0.,0.,-1.));
#16293=DIRECTION('center_axis',(-1.,0.,0.));
#16294=DIRECTION('ref_axis',(0.,-2.96059473233375E-15,-1.));
#16295=DIRECTION('',(-1.,0.,0.));
#16296=DIRECTION('center_axis',(0.,1.,0.));
#16297=DIRECTION('ref_axis',(0.,0.,-1.));
#16298=DIRECTION('',(0.,0.,1.));
#16299=DIRECTION('center_axis',(0.,0.,1.));
#16300=DIRECTION('ref_axis',(0.70710678118654,0.707106781186555,0.));
#16301=DIRECTION('center_axis',(0.,-1.,0.));
#16302=DIRECTION('ref_axis',(-0.70710678118654,0.,-0.707106781186555));
#22641=CARTESIAN_POINT('',(0.,0.,0.));
#22642=CARTESIAN_POINT('Ctrl Pts',(-67.9629497348173,6.06724190764723,-107.927825300627));
#22643=CARTESIAN_POINT('Ctrl Pts',(-67.9731885875005,6.09608154848999,-107.930287524609));
#22644=CARTESIAN_POINT('Ctrl Pts',(-68.0649619777051,6.35254287993133,-107.950374147766));
#22645=CARTESIAN_POINT('Ctrl Pts',(-68.1421523199026,6.56142467898147,-107.95));
#22646=CARTESIAN_POINT('Ctrl Pts',(-68.15,6.58309518948455,-107.95));
#22647=CARTESIAN_POINT('Ctrl Pts',(-68.0878080075958,6.02164898271821,-107.935082546577));
#22648=CARTESIAN_POINT('Ctrl Pts',(-68.0951549181554,6.04220422326524,-107.936123736671));
#22649=CARTESIAN_POINT('Ctrl Pts',(-68.1598746388879,6.22406166120123,-107.952418698047));
#22650=CARTESIAN_POINT('Ctrl Pts',(-68.2153859993183,6.37331286135221,-107.95));
#22651=CARTESIAN_POINT('Ctrl Pts',(-68.220972086323,6.38873012632303,-107.95));
#22652=CARTESIAN_POINT('Ctrl Pts',(-68.2126662803743,5.97605605778919,-107.942339792527));
#22653=CARTESIAN_POINT('Ctrl Pts',(-68.2170579361042,5.98825113903969,-107.942573272401));
#22654=CARTESIAN_POINT('Ctrl Pts',(-68.256721155555,6.09746416349077,-107.947668564864));
#22655=CARTESIAN_POINT('Ctrl Pts',(-68.288619678734,6.18520104372295,-107.95));
#22656=CARTESIAN_POINT('Ctrl Pts',(-68.291944172646,6.19436506316152,-107.95));
#22657=CARTESIAN_POINT('Ctrl Pts',(-68.3375245531529,5.93046313286018,-107.949597038478));
#22658=CARTESIAN_POINT('Ctrl Pts',(-68.3389416671525,5.93434379913925,-107.949642016394));
#22659=CARTESIAN_POINT('Ctrl Pts',(-68.351571877404,5.96893138250399,-107.950007869635));
#22660=CARTESIAN_POINT('Ctrl Pts',(-68.3618533581497,5.9970892260937,-107.95));
#22661=CARTESIAN_POINT('Ctrl Pts',(-68.3629162589689,6.,-107.95));
#22662=CARTESIAN_POINT('',(-68.15,6.58309518948455,-107.95));
#22663=CARTESIAN_POINT('',(-67.9629497348173,6.06724190764723,-107.927825300627));
#22664=CARTESIAN_POINT('Ctrl Pts',(-68.15,6.58309518948455,-107.95));
#22665=CARTESIAN_POINT('Ctrl Pts',(-68.1494585269681,6.58159997091316,-107.95));
#22666=CARTESIAN_POINT('Ctrl Pts',(-68.1489155383018,6.58010061545652,-107.949999490713));
#22667=CARTESIAN_POINT('Ctrl Pts',(-68.1483145418233,6.57844322897782,-107.949998224517));
#22668=CARTESIAN_POINT('Ctrl Pts',(-68.1476856008723,6.57670877916767,-107.949996899447));
#22669=CARTESIAN_POINT('Ctrl Pts',(-68.1469931402562,6.57480128397559,-107.949994750064));
#22670=CARTESIAN_POINT('Ctrl Pts',(-68.1461923150497,6.57259867099725,-107.949990938408));
#22671=CARTESIAN_POINT('Ctrl Pts',(-68.14536192547,6.57031474330575,-107.949986986036));
#22672=CARTESIAN_POINT('Ctrl Pts',(-68.1444150906044,6.56771369413093,-107.949981251966));
#22673=CARTESIAN_POINT('Ctrl Pts',(-68.1433221006719,6.56471475376682,-107.949972128052));
#22674=CARTESIAN_POINT('Ctrl Pts',(-68.1421797916733,6.56158049199336,-107.949962592439));
#22675=CARTESIAN_POINT('Ctrl Pts',(-68.1408779237317,6.55801185344092,-107.949949350216));
#22676=CARTESIAN_POINT('Ctrl Pts',(-68.1394032019918,6.55397281294346,-107.949929814341));
#22677=CARTESIAN_POINT('Ctrl Pts',(-68.1378429799736,6.54969960007502,-107.949909145831));
#22678=CARTESIAN_POINT('Ctrl Pts',(-68.1360893891363,6.54490016320098,-107.94988140751));
#22679=CARTESIAN_POINT('Ctrl Pts',(-68.1341478192351,6.53958932246212,-107.949842927308));
#22680=CARTESIAN_POINT('Ctrl Pts',(-68.1320491206422,6.53384868238592,-107.949801332955));
#22681=CARTESIAN_POINT('Ctrl Pts',(-68.1297309447041,6.52751095521807,-107.949747125478));
#22682=CARTESIAN_POINT('Ctrl Pts',(-68.1272221189739,6.52065461386469,-107.949675664339));
#22683=CARTESIAN_POINT('Ctrl Pts',(-68.1243771906191,6.51287974146469,-107.949594629686));
#22684=CARTESIAN_POINT('Ctrl Pts',(-68.1212873988534,6.50443878957247,-107.94949126786));
#22685=CARTESIAN_POINT('Ctrl Pts',(-68.1180187985553,6.49551117516029,-107.949360496118));
#22686=CARTESIAN_POINT('Ctrl Pts',(-68.1129443811809,6.48165128482386,-107.949157476373));
#22687=CARTESIAN_POINT('Ctrl Pts',(-68.1074407974137,6.46662336130254,-107.948887112081));
#22688=CARTESIAN_POINT('Ctrl Pts',(-68.1018027325981,6.45122664552437,-107.948546819801));
#22689=CARTESIAN_POINT('Ctrl Pts',(-68.0982065867868,6.44140610660473,-107.948329770034));
#22690=CARTESIAN_POINT('Ctrl Pts',(-68.0945567798222,6.43143836252592,-107.948084794035));
#22691=CARTESIAN_POINT('Ctrl Pts',(-68.0909213073327,6.42150762201437,-107.947815585253));
#22692=CARTESIAN_POINT('Ctrl Pts',(-68.0875130518738,6.4121975527848,-107.94756320202));
#22693=CARTESIAN_POINT('Ctrl Pts',(-68.0841178949647,6.40292137962132,-107.947289665233));
#22694=CARTESIAN_POINT('Ctrl Pts',(-68.0807745846575,6.39378372955142,-107.946999273444));
#22695=CARTESIAN_POINT('Ctrl Pts',(-68.0778535573511,6.38580022729814,-107.946745560128));
#22696=CARTESIAN_POINT('Ctrl Pts',(-68.0749721054198,6.37792247617486,-107.946479072676));
#22697=CARTESIAN_POINT('Ctrl Pts',(-68.0721398855605,6.37017591351234,-107.94620211164));
#22698=CARTESIAN_POINT('Ctrl Pts',(-68.069478336024,6.36289616077843,-107.945941840349));
#22699=CARTESIAN_POINT('Ctrl Pts',(-68.0668603435943,6.35573249576057,-107.945672384873));
#22700=CARTESIAN_POINT('Ctrl Pts',(-68.0642778922634,6.34866190828134,-107.945394066011));
#22701=CARTESIAN_POINT('Ctrl Pts',(-68.061799072167,6.34187505653043,-107.945126915811));
#22702=CARTESIAN_POINT('Ctrl Pts',(-68.0593530791771,6.3351742015672,-107.944851655774));
#22703=CARTESIAN_POINT('Ctrl Pts',(-68.0569163899697,6.32849354472908,-107.944566197081));
#22704=CARTESIAN_POINT('Ctrl Pts',(-68.0544290695812,6.32167407267163,-107.944274806934));
#22705=CARTESIAN_POINT('Ctrl Pts',(-68.0519486504824,6.314867926326,-107.943972484575));
#22706=CARTESIAN_POINT('Ctrl Pts',(-68.0494441127739,6.30798832458315,-107.943655160346));
#22707=CARTESIAN_POINT('Ctrl Pts',(-68.0468597289661,6.30088939718941,-107.943327719639));
#22708=CARTESIAN_POINT('Ctrl Pts',(-68.044249738723,6.29371244739674,-107.942984257085));
#22709=CARTESIAN_POINT('Ctrl Pts',(-68.0416004982127,6.286418578412,-107.9426219452));
#22710=CARTESIAN_POINT('Ctrl Pts',(-68.0388040332892,6.27871937228366,-107.942239498806));
#22711=CARTESIAN_POINT('Ctrl Pts',(-68.0359639561777,6.27089020577216,-107.941835999561));
#22712=CARTESIAN_POINT('Ctrl Pts',(-68.0330849632465,6.26294290518048,-107.941410686168));
#22713=CARTESIAN_POINT('Ctrl Pts',(-68.029986346019,6.2543893438785,-107.940952927695));
#22714=CARTESIAN_POINT('Ctrl Pts',(-68.0268428260038,6.24569938969678,-107.940469835404));
#22715=CARTESIAN_POINT('Ctrl Pts',(-68.0236813969289,6.23694695262799,-107.939964309648));
#22716=CARTESIAN_POINT('Ctrl Pts',(-68.0201202563992,6.22708791178246,-107.939394868356));
#22717=CARTESIAN_POINT('Ctrl Pts',(-68.0165366962784,6.21715035833223,-107.938796864838));
#22718=CARTESIAN_POINT('Ctrl Pts',(-68.0129916053749,6.20730341158762,-107.938180626381));
#22719=CARTESIAN_POINT('Ctrl Pts',(-68.0063167094922,6.18876302825924,-107.937020338068));
#22720=CARTESIAN_POINT('Ctrl Pts',(-67.9997811710551,6.17055030095131,-107.935793011526));
#22721=CARTESIAN_POINT('Ctrl Pts',(-67.9938677249504,6.15402777629214,-107.934616283726));
#22722=CARTESIAN_POINT('Ctrl Pts',(-67.9908424118573,6.14557486925642,-107.934014270964));
#22723=CARTESIAN_POINT('Ctrl Pts',(-67.9879803302263,6.13756600214908,-107.933426406399));
#22724=CARTESIAN_POINT('Ctrl Pts',(-67.9853349496579,6.13015493599242,-107.93286998997));
#22725=CARTESIAN_POINT('Ctrl Pts',(-67.9829511051419,6.12347656629908,-107.932368583757));
#22726=CARTESIAN_POINT('Ctrl Pts',(-67.9807434357073,6.11728427347295,-107.931892853576));
#22727=CARTESIAN_POINT('Ctrl Pts',(-67.9787370277375,6.11165176399922,-107.931453129965));
#22728=CARTESIAN_POINT('Ctrl Pts',(-67.9768605583099,6.10638402583844,-107.931041883635));
#22729=CARTESIAN_POINT('Ctrl Pts',(-67.9751602598371,6.10160632696771,-107.930662212486));
#22730=CARTESIAN_POINT('Ctrl Pts',(-67.973641409216,6.09733604160012,-107.930318939573));
#22731=CARTESIAN_POINT('Ctrl Pts',(-67.9722286436796,6.09336401702179,-107.929999642775));
#22732=CARTESIAN_POINT('Ctrl Pts',(-67.9709728991424,6.08983111529492,-107.92971186547));
#22733=CARTESIAN_POINT('Ctrl Pts',(-67.9698637164228,6.08670954431878,-107.929455527493));
#22734=CARTESIAN_POINT('Ctrl Pts',(-67.9687881735891,6.08368264601479,-107.929206963871));
#22735=CARTESIAN_POINT('Ctrl Pts',(-67.9678505353126,6.0810427906326,-107.928987991027));
#22736=CARTESIAN_POINT('Ctrl Pts',(-67.9670258484074,6.07872068925269,-107.928794234602));
#22737=CARTESIAN_POINT('Ctrl Pts',(-67.9662228305955,6.07645960233928,-107.928605569231));
#22738=CARTESIAN_POINT('Ctrl Pts',(-67.965526990813,6.07450002928015,-107.92844082974));
#22739=CARTESIAN_POINT('Ctrl Pts',(-67.9648991159876,6.07273187235018,-107.928291502419));
#22740=CARTESIAN_POINT('Ctrl Pts',(-67.9642908646836,6.07101897717607,-107.928146842155));
#22741=CARTESIAN_POINT('Ctrl Pts',(-67.9637464441481,6.06948585391573,-107.928016653354));
#22742=CARTESIAN_POINT('Ctrl Pts',(-67.9632138925135,6.06798592939913,-107.927888777429));
#22743=CARTESIAN_POINT('Ctrl Pts',(-67.9631256466347,6.06773738606814,-107.927867587891));
#22744=CARTESIAN_POINT('Ctrl Pts',(-67.9630376883609,6.06748964522963,-107.927846451563));
#22745=CARTESIAN_POINT('Ctrl Pts',(-67.9629497348173,6.06724190764723,-107.927825300627));
#22746=CARTESIAN_POINT('',(-68.3375245531529,5.93046313286018,-107.949597038478));
#22747=CARTESIAN_POINT('Ctrl Pts',(-68.3375245531529,5.93046313286018,-107.949597038478));
#22748=CARTESIAN_POINT('Ctrl Pts',(-68.2126662803743,5.97605605778919,-107.942339792527));
#22749=CARTESIAN_POINT('Ctrl Pts',(-68.0878080075958,6.02164898271821,-107.935082546577));
#22750=CARTESIAN_POINT('Ctrl Pts',(-67.9629497348173,6.06724190764723,-107.927825300627));
#22751=CARTESIAN_POINT('',(-68.3629162589689,6.,-107.95));
#22752=CARTESIAN_POINT('Ctrl Pts',(-68.3375245531529,5.93046313286018,-107.949597038478));
#22753=CARTESIAN_POINT('Ctrl Pts',(-68.3376484128971,5.9308023139938,-107.949600969674));
#22754=CARTESIAN_POINT('Ctrl Pts',(-68.3377738812747,5.93114590045188,-107.949604929021));
#22755=CARTESIAN_POINT('Ctrl Pts',(-68.3379336160622,5.93158332280906,-107.949609917176));
#22756=CARTESIAN_POINT('Ctrl Pts',(-68.3381007845541,5.93204110183711,-107.949615137469));
#22757=CARTESIAN_POINT('Ctrl Pts',(-68.3383053431287,5.93260127070113,-107.949621481053));
#22758=CARTESIAN_POINT('Ctrl Pts',(-68.3385647351012,5.93331159796506,-107.949629376639));
#22759=CARTESIAN_POINT('Ctrl Pts',(-68.3388581498122,5.93411509418272,-107.949638307837));
#22760=CARTESIAN_POINT('Ctrl Pts',(-68.3392217164581,5.93511069785869,-107.949649222747));
#22761=CARTESIAN_POINT('Ctrl Pts',(-68.3396564658575,5.93630123568428,-107.949661862757));
#22762=CARTESIAN_POINT('Ctrl Pts',(-68.3401321391992,5.93760384152248,-107.9496756926));
#22763=CARTESIAN_POINT('Ctrl Pts',(-68.3406925812451,5.93913858691483,-107.94969155866));
#22764=CARTESIAN_POINT('Ctrl Pts',(-68.3413155502779,5.94084456975624,-107.949708379169));
#22765=CARTESIAN_POINT('Ctrl Pts',(-68.3422472252028,5.94339593483566,-107.949733534908));
#22766=CARTESIAN_POINT('Ctrl Pts',(-68.3433170705235,5.94632569724319,-107.949760665181));
#22767=CARTESIAN_POINT('Ctrl Pts',(-68.3444107004731,5.94932062429725,-107.949785962922));
#22768=CARTESIAN_POINT('Ctrl Pts',(-68.3451482244235,5.95134034809204,-107.949803023254));
#22769=CARTESIAN_POINT('Ctrl Pts',(-68.3458954545405,5.95338666559863,-107.949819263662));
#22770=CARTESIAN_POINT('Ctrl Pts',(-68.3466257052537,5.95538649749514,-107.94983413399));
#22771=CARTESIAN_POINT('Ctrl Pts',(-68.3472620357263,5.95712912362719,-107.949847091791));
#22772=CARTESIAN_POINT('Ctrl Pts',(-68.3478852316262,5.9588357900753,-107.949859020331));
#22773=CARTESIAN_POINT('Ctrl Pts',(-68.3484914174909,5.96049588209922,-107.949869950646));
#22774=CARTESIAN_POINT('Ctrl Pts',(-68.3490583868923,5.96204857647187,-107.949880173838));
#22775=CARTESIAN_POINT('Ctrl Pts',(-68.3496102870568,5.9635600102806,-107.949889531659));
#22776=CARTESIAN_POINT('Ctrl Pts',(-68.3501598186094,5.96506496295212,-107.949898294404));
#22777=CARTESIAN_POINT('Ctrl Pts',(-68.3507102523001,5.96657238622828,-107.949907071534));
#22778=CARTESIAN_POINT('Ctrl Pts',(-68.3512614068472,5.96808178899628,-107.949915301922));
#22779=CARTESIAN_POINT('Ctrl Pts',(-68.351827369383,5.96963174796697,-107.949923146947));
#22780=CARTESIAN_POINT('Ctrl Pts',(-68.3524400984799,5.97130978299589,-107.949931640221));
#22781=CARTESIAN_POINT('Ctrl Pts',(-68.3530700019396,5.97303485537861,-107.949939665741));
#22782=CARTESIAN_POINT('Ctrl Pts',(-68.3537140997498,5.9747988021213,-107.949947074735));
#22783=CARTESIAN_POINT('Ctrl Pts',(-68.3544669504786,5.97686058306484,-107.949955734703));
#22784=CARTESIAN_POINT('Ctrl Pts',(-68.3552388966772,5.97897466126154,-107.949963524226));
#22785=CARTESIAN_POINT('Ctrl Pts',(-68.35600106939,5.98106197314171,-107.94997011252));
#22786=CARTESIAN_POINT('Ctrl Pts',(-68.3569159942254,5.98356761713371,-107.949978021219));
#22787=CARTESIAN_POINT('Ctrl Pts',(-68.3578152161114,5.98603025599149,-107.949984153345));
#22788=CARTESIAN_POINT('Ctrl Pts',(-68.3586312279608,5.98826500948253,-107.949988524155));
#22789=CARTESIAN_POINT('Ctrl Pts',(-68.3592601969867,5.98998752212431,-107.949991893107));
#22790=CARTESIAN_POINT('Ctrl Pts',(-68.3598389431586,5.9915724906411,-107.949994240505));
#22791=CARTESIAN_POINT('Ctrl Pts',(-68.3603434552782,5.99295415655121,-107.949995863006));
#22792=CARTESIAN_POINT('Ctrl Pts',(-68.360801738962,5.99420922044048,-107.949997336838));
#22793=CARTESIAN_POINT('Ctrl Pts',(-68.3611984503128,5.99529565802497,-107.949998223794));
#22794=CARTESIAN_POINT('Ctrl Pts',(-68.3615283752455,5.99619919007954,-107.949998796154));
#22795=CARTESIAN_POINT('Ctrl Pts',(-68.3618379571857,5.99704701083741,-107.949999333221));
#22796=CARTESIAN_POINT('Ctrl Pts',(-68.3620885335494,5.99773323519729,-107.94999959747));
#22797=CARTESIAN_POINT('Ctrl Pts',(-68.3622911398108,5.99828808589258,-107.949999755779));
#22798=CARTESIAN_POINT('Ctrl Pts',(-68.3624807303376,5.99880729213499,-107.949999903919));
#22799=CARTESIAN_POINT('Ctrl Pts',(-68.3626282304674,5.99921122722297,-107.949999958751));
#22800=CARTESIAN_POINT('Ctrl Pts',(-68.3627584528728,5.99956784464617,-107.949999984437));
#22801=CARTESIAN_POINT('Ctrl Pts',(-68.3628129524334,5.99971709310149,-107.949999995187));
#22802=CARTESIAN_POINT('Ctrl Pts',(-68.3628646310546,5.99985861598442,-107.95));
#22803=CARTESIAN_POINT('Ctrl Pts',(-68.3629162589689,6.,-107.95));
#22804=CARTESIAN_POINT('',(-68.2564581294845,6.29154759474227,-107.95));
#22805=CARTESIAN_POINT('Ctrl Pts',(-68.3375240385289,0.000402977856687192,
-102.019538276432));
#22806=CARTESIAN_POINT('Ctrl Pts',(-68.3380554670653,0.000386110454297121,
-102.01808299709));
#22807=CARTESIAN_POINT('Ctrl Pts',(-68.3397274021881,0.00032759961132862,
-102.013504598476));
#22808=CARTESIAN_POINT('Ctrl Pts',(-68.3466614877139,0.000156761636871131,
-101.994515645545));
#22809=CARTESIAN_POINT('Ctrl Pts',(-68.3522721650115,5.98098402742648E-5,
-101.979150165178));
#22810=CARTESIAN_POINT('Ctrl Pts',(-68.3583205753897,7.84684658830335E-6,
-101.962585741651));
#22811=CARTESIAN_POINT('Ctrl Pts',(-68.3618857180998,-2.66424903465483E-7,
-101.95282217754));
#22812=CARTESIAN_POINT('Ctrl Pts',(-68.3625619515145,-3.08148791101958E-32,
-101.950970277635));
#22813=CARTESIAN_POINT('Ctrl Pts',(-68.3629162589689,-3.08148791101958E-32,
-101.95));
#22814=CARTESIAN_POINT('Ctrl Pts',(-68.2126657709715,0.00766025835870256,
-101.973945350221));
#22815=CARTESIAN_POINT('Ctrl Pts',(-68.2143126524885,0.00757270097272666,
-101.969372165137));
#22816=CARTESIAN_POINT('Ctrl Pts',(-68.22076700718,0.00689140766747181,
-101.951555360678));
#22817=CARTESIAN_POINT('Ctrl Pts',(-68.239810705309,0.00496924519147893,
-101.899128861556));
#22818=CARTESIAN_POINT('Ctrl Pts',(-68.2597635158947,0.00276030806902361,
-101.844195710985));
#22819=CARTESIAN_POINT('Ctrl Pts',(-68.2772007293579,0.00110275965346496,
-101.796221353378));
#22820=CARTESIAN_POINT('Ctrl Pts',(-68.2878618278732,0.000211776221296321,
-101.76688366558));
#22821=CARTESIAN_POINT('Ctrl Pts',(-68.2908360008298,1.38777878078145E-16,
-101.758689629699));
#22822=CARTESIAN_POINT('Ctrl Pts',(-68.291944172646,1.38777878078145E-16,
-101.755634936838));
#22823=CARTESIAN_POINT('Ctrl Pts',(-68.0878075034141,0.0149175388607179,
-101.92835242401));
#22824=CARTESIAN_POINT('Ctrl Pts',(-68.0905626050853,0.0145270867471023,
-101.920644179277));
#22825=CARTESIAN_POINT('Ctrl Pts',(-68.098117885938,0.012488559345189,-101.899889546156));
#22826=CARTESIAN_POINT('Ctrl Pts',(-68.1376182455488,0.00738521760650383,
-101.792512628689));
#22827=CARTESIAN_POINT('Ctrl Pts',(-68.1645278494201,0.00313818569707965,
-101.718138514254));
#22828=CARTESIAN_POINT('Ctrl Pts',(-68.1976204498916,0.00103052104806465,
-101.626708713674));
#22829=CARTESIAN_POINT('Ctrl Pts',(-68.2165346834987,0.000408528025162008,
-101.573838723558));
#22830=CARTESIAN_POINT('Ctrl Pts',(-68.219110050145,2.77555756156289E-16,
-101.566408981763));
#22831=CARTESIAN_POINT('Ctrl Pts',(-68.220972086323,2.77555756156289E-16,
-101.561269873677));
#22832=CARTESIAN_POINT('Ctrl Pts',(-67.9629492358567,0.0221748193627333,
-101.882759497799));
#22833=CARTESIAN_POINT('Ctrl Pts',(-67.9667888156613,0.0212514803473293,
-101.871944602866));
#22834=CARTESIAN_POINT('Ctrl Pts',(-67.9787772078244,0.0180626748813272,
-101.837962280823));
#22835=CARTESIAN_POINT('Ctrl Pts',(-68.0292947457965,0.00869185796202674,
-101.697150420595));
#22836=CARTESIAN_POINT('Ctrl Pts',(-68.0708521582608,0.00330806576115239,
-101.583201284989));
#22837=CARTESIAN_POINT('Ctrl Pts',(-68.1158766125516,0.000432114042481723,
-101.460351904441));
#22838=CARTESIAN_POINT('Ctrl Pts',(-68.1423791757427,-1.45647633857201E-5,
-101.387901818545));
#22839=CARTESIAN_POINT('Ctrl Pts',(-68.1473840994603,4.16333634234434E-16,
-101.374128333826));
#22840=CARTESIAN_POINT('Ctrl Pts',(-68.15,4.16333634234434E-16,-101.366904810515));
#22841=CARTESIAN_POINT('',(-68.3629162589689,0.,-101.95));
#22842=CARTESIAN_POINT('',(-68.3375240385289,0.000402977856687192,-102.019538276432));
#22843=CARTESIAN_POINT('Ctrl Pts',(-68.3629162589689,0.,-101.95));
#22844=CARTESIAN_POINT('Ctrl Pts',(-68.3627923897953,0.,-101.950339218064));
#22845=CARTESIAN_POINT('Ctrl Pts',(-68.3626669120248,2.29080291819244E-8,
-101.950682841491));
#22846=CARTESIAN_POINT('Ctrl Pts',(-68.3625071684643,1.04590663241311E-7,
-101.951120307079));
#22847=CARTESIAN_POINT('Ctrl Pts',(-68.3623399907767,1.90074634203094E-7,
-101.95157813139));
#22848=CARTESIAN_POINT('Ctrl Pts',(-68.3621354236744,3.38991582082524E-7,
-101.952138352405));
#22849=CARTESIAN_POINT('Ctrl Pts',(-68.3618760240636,6.76277169375794E-7,
-101.952848741051));
#22850=CARTESIAN_POINT('Ctrl Pts',(-68.3615826009174,1.05780202161708E-6,
-101.953652306139));
#22851=CARTESIAN_POINT('Ctrl Pts',(-68.3612190270723,1.68218512989849E-6,
-101.954647990211));
#22852=CARTESIAN_POINT('Ctrl Pts',(-68.3607842715223,2.84078836632062E-6,
-101.955838617329));
#22853=CARTESIAN_POINT('Ctrl Pts',(-68.3603085925965,4.1084504882767E-6,
-101.957141317729));
#22854=CARTESIAN_POINT('Ctrl Pts',(-68.359748146621,6.0304302990709E-6,
-101.958676166968));
#22855=CARTESIAN_POINT('Ctrl Pts',(-68.3591251743955,8.98260877768564E-6,
-101.960382255277));
#22856=CARTESIAN_POINT('Ctrl Pts',(-68.3581934848705,1.33977554757658E-5,
-101.962933804996));
#22857=CARTESIAN_POINT('Ctrl Pts',(-68.3571236235583,2.02240548300365E-5,
-101.965863762444));
#22858=CARTESIAN_POINT('Ctrl Pts',(-68.3560299762102,2.96381295097348E-5,
-101.968858861994));
#22859=CARTESIAN_POINT('Ctrl Pts',(-68.3552924432318,3.59867852697833E-5,
-101.970878694707));
#22860=CARTESIAN_POINT('Ctrl Pts',(-68.3545452035351,4.34635720193775E-5,
-101.97292511089));
#22861=CARTESIAN_POINT('Ctrl Pts',(-68.3538149425036,5.1771638321263E-5,
-101.974925027172));
#22862=CARTESIAN_POINT('Ctrl Pts',(-68.3531786038672,5.90111641261043E-5,
-101.976667724572));
#22863=CARTESIAN_POINT('Ctrl Pts',(-68.3525553992048,6.68631533653939E-5,
-101.978374451692));
#22864=CARTESIAN_POINT('Ctrl Pts',(-68.3519492040121,7.51735369854956E-5,
-101.980034593268));
#22865=CARTESIAN_POINT('Ctrl Pts',(-68.3513822292988,8.29462435779145E-5,
-101.981587324641));
#22866=CARTESIAN_POINT('Ctrl Pts',(-68.3508303231258,9.11060791431646E-5,
-101.983098786388));
#22867=CARTESIAN_POINT('Ctrl Pts',(-68.350280785426,9.97858279365715E-5,
-101.984603756704));
#22868=CARTESIAN_POINT('Ctrl Pts',(-68.3497303427571,0.000108479870387661,
-101.986111205378));
#22869=CARTESIAN_POINT('Ctrl Pts',(-68.3491791791713,0.000117743553775951,
-101.987620623011));
#22870=CARTESIAN_POINT('Ctrl Pts',(-68.3486132068006,0.000127862609702767,
-101.989170588042));
#22871=CARTESIAN_POINT('Ctrl Pts',(-68.3480004704559,0.000138817761689317,
-101.990848620322));
#22872=CARTESIAN_POINT('Ctrl Pts',(-68.3473705590191,0.000150785773284043,
-101.992573678939));
#22873=CARTESIAN_POINT('Ctrl Pts',(-68.3467264521374,0.000163820817507876,
-101.994337602245));
#22874=CARTESIAN_POINT('Ctrl Pts',(-68.3459735972113,0.000179056638668035,
-101.996399338252));
#22875=CARTESIAN_POINT('Ctrl Pts',(-68.3452016456489,0.00019576893702528,
-101.998513357157));
#22876=CARTESIAN_POINT('Ctrl Pts',(-68.3444394655154,0.00021337221006501,
-102.000600602695));
#22877=CARTESIAN_POINT('Ctrl Pts',(-68.3435245038817,0.000234504116753176,
-102.003106243427));
#22878=CARTESIAN_POINT('Ctrl Pts',(-68.3426252430714,0.000256914204160928,
-102.005568866458));
#22879=CARTESIAN_POINT('Ctrl Pts',(-68.3418091957487,0.000278444425536151,
-102.007803594829));
#22880=CARTESIAN_POINT('Ctrl Pts',(-68.3411802068165,0.000295039383418406,
-102.009526067744));
#22881=CARTESIAN_POINT('Ctrl Pts',(-68.3406014416822,0.000311061775608003,
-102.011110994502));
#22882=CARTESIAN_POINT('Ctrl Pts',(-68.340096913208,0.000325452808408677,
-102.012492621815));
#22883=CARTESIAN_POINT('Ctrl Pts',(-68.3396386155056,0.000338525167266646,
-102.013747648352));
#22884=CARTESIAN_POINT('Ctrl Pts',(-68.3392418920764,0.000350230045051696,
-102.014834051977));
#22885=CARTESIAN_POINT('Ctrl Pts',(-68.338911958005,0.000360129655326169,
-102.015737555252));
#22886=CARTESIAN_POINT('Ctrl Pts',(-68.338602367729,0.000369418853813961,
-102.01658534835));
#22887=CARTESIAN_POINT('Ctrl Pts',(-68.338351785533,0.00037710798045477,
-102.017271549939));
#22888=CARTESIAN_POINT('Ctrl Pts',(-68.33814917651,0.000383380404201716,
-102.017826380339));
#22889=CARTESIAN_POINT('Ctrl Pts',(-68.3379595836666,0.000389249869614026,
-102.018345566857));
#22890=CARTESIAN_POINT('Ctrl Pts',(-68.3378120837904,0.000393876634263669,
-102.018749484727));
#22891=CARTESIAN_POINT('Ctrl Pts',(-68.3376818644882,0.00039798407021685,
-102.019106081145));
#22892=CARTESIAN_POINT('Ctrl Pts',(-68.3376273573398,0.000399703359268928,
-102.019255345145));
#22893=CARTESIAN_POINT('Ctrl Pts',(-68.3375756725639,0.000401339005957926,
-102.01939688029));
#22894=CARTESIAN_POINT('Ctrl Pts',(-68.3375240385289,0.000402977856687414,
-102.019538276432));
#22895=CARTESIAN_POINT('',(-67.9629492358567,0.0221748193627333,-101.882759497799));
#22896=CARTESIAN_POINT('Ctrl Pts',(-67.9629492358567,0.0221748193627333,
-101.882759497799));
#22897=CARTESIAN_POINT('Ctrl Pts',(-68.0878075034141,0.0149175388607179,
-101.92835242401));
#22898=CARTESIAN_POINT('Ctrl Pts',(-68.2126657709715,0.00766025835870256,
-101.973945350221));
#22899=CARTESIAN_POINT('Ctrl Pts',(-68.3375240385289,0.000402977856687192,
-102.019538276432));
#22900=CARTESIAN_POINT('',(-68.15,4.16333634234434E-16,-101.366904810515));
#22901=CARTESIAN_POINT('Ctrl Pts',(-67.9629492358567,0.0221748193627326,
-101.882759497799));
#22902=CARTESIAN_POINT('Ctrl Pts',(-67.963479204653,0.0220473728994396,
-101.881266741523));
#22903=CARTESIAN_POINT('Ctrl Pts',(-67.9640107571927,0.0219200770074053,
-101.879769844391));
#22904=CARTESIAN_POINT('Ctrl Pts',(-67.9645984647885,0.0217800627449767,
-101.878114792924));
#22905=CARTESIAN_POINT('Ctrl Pts',(-67.9652135065934,0.0216335364361574,
-101.876382765213));
#22906=CARTESIAN_POINT('Ctrl Pts',(-67.9658900396362,0.0214730787737821,
-101.874477552795));
#22907=CARTESIAN_POINT('Ctrl Pts',(-67.9666715313617,0.0212890956287135,
-101.872276993515));
#22908=CARTESIAN_POINT('Ctrl Pts',(-67.9674818862734,0.0210983173512174,
-101.869995159986));
#22909=CARTESIAN_POINT('Ctrl Pts',(-67.9684050288704,0.0208822544197106,
-101.867395949033));
#22910=CARTESIAN_POINT('Ctrl Pts',(-67.9694699998139,0.0206355672518712,
-101.864398540544));
#22911=CARTESIAN_POINT('Ctrl Pts',(-67.9705830508428,0.0203777429350113,
-101.861265808498));
#22912=CARTESIAN_POINT('Ctrl Pts',(-67.9718509454421,0.0200864902186626,
-101.857698345532));
#22913=CARTESIAN_POINT('Ctrl Pts',(-67.9732871132033,0.0197612188310728,
-101.853660121473));
#22914=CARTESIAN_POINT('Ctrl Pts',(-67.9748066016365,0.0194170765069945,
-101.849387615911));
#22915=CARTESIAN_POINT('Ctrl Pts',(-67.9765143547195,0.0190349035407727,
-101.844588446135));
#22916=CARTESIAN_POINT('Ctrl Pts',(-67.9784060294671,0.0186194849647396,
-101.839277485123));
#22917=CARTESIAN_POINT('Ctrl Pts',(-67.980450937861,0.0181704157290355,
-101.833536313833));
#22918=CARTESIAN_POINT('Ctrl Pts',(-67.9827106320596,0.0176825934726907,
-101.827197519925));
#22919=CARTESIAN_POINT('Ctrl Pts',(-67.9851583897371,0.0171671675728304,
-101.820339719563));
#22920=CARTESIAN_POINT('Ctrl Pts',(-67.9879348778888,0.0165825206867542,
-101.812560926087));
#22921=CARTESIAN_POINT('Ctrl Pts',(-67.9909530856542,0.0159625611116039,
-101.80411516068));
#22922=CARTESIAN_POINT('Ctrl Pts',(-67.9941504668417,0.0153275058890211,
-101.795182272282));
#22923=CARTESIAN_POINT('Ctrl Pts',(-67.999103381522,0.0143437713418104,
-101.781344749796));
#22924=CARTESIAN_POINT('Ctrl Pts',(-68.0044847691745,0.013325450983196,
-101.76634326983));
#22925=CARTESIAN_POINT('Ctrl Pts',(-68.0100131590849,0.0123429144795248,
-101.750973409286));
#22926=CARTESIAN_POINT('Ctrl Pts',(-68.0135448047949,0.0117152505693476,
-101.741154835898));
#22927=CARTESIAN_POINT('Ctrl Pts',(-68.0171353174443,0.0111019329412723,
-101.731188757335));
#22928=CARTESIAN_POINT('Ctrl Pts',(-68.0207185807078,0.0105151587105776,
-101.721259398455));
#22929=CARTESIAN_POINT('Ctrl Pts',(-68.0240778900172,0.00996505786930133,
-101.711950624506));
#22930=CARTESIAN_POINT('Ctrl Pts',(-68.0274303123987,0.00943826307777242,
-101.702675497437));
#22931=CARTESIAN_POINT('Ctrl Pts',(-68.030737812301,0.00893961634699059,
-101.693538665169));
#22932=CARTESIAN_POINT('Ctrl Pts',(-68.0336280436274,0.00850387804171688,
-101.685554520158));
#22933=CARTESIAN_POINT('Ctrl Pts',(-68.0364839523172,0.00808954505312252,
-101.677675989526));
#22934=CARTESIAN_POINT('Ctrl Pts',(-68.0392959553743,0.00769663985092728,
-101.669928535905));
#22935=CARTESIAN_POINT('Ctrl Pts',(-68.0419389442863,0.00732735003445809,
-101.662646739406));
#22936=CARTESIAN_POINT('Ctrl Pts',(-68.0445430543738,0.00697694539912664,
-101.655480972348));
#22937=CARTESIAN_POINT('Ctrl Pts',(-68.047116215687,0.00664325368379659,
-101.648408198893));
#22938=CARTESIAN_POINT('Ctrl Pts',(-68.0495855904285,0.00632302117871791,
-101.641620700561));
#22939=CARTESIAN_POINT('Ctrl Pts',(-68.0520263717414,0.00601814482450214,
-101.634919083727));
#22940=CARTESIAN_POINT('Ctrl Pts',(-68.0544620138332,0.0057251777884475,
-101.628237508679));
#22941=CARTESIAN_POINT('Ctrl Pts',(-68.0569473578203,0.00542623244506826,
-101.62141958891));
#22942=CARTESIAN_POINT('Ctrl Pts',(-68.0594301387455,0.00513933042164893,
-101.61461481663));
#22943=CARTESIAN_POINT('Ctrl Pts',(-68.0619414059947,0.00486121713136911,
-101.607736477541));
#22944=CARTESIAN_POINT('Ctrl Pts',(-68.0645328639825,0.00457422302197651,
-101.600638496719));
#22945=CARTESIAN_POINT('Ctrl Pts',(-68.0671545943895,0.00429665256098612,
-101.593462367059));
#22946=CARTESIAN_POINT('Ctrl Pts',(-68.069820349461,0.00402812635154237,
-101.586169212969));
#22947=CARTESIAN_POINT('Ctrl Pts',(-68.0726342429012,0.0037446779029668,
-101.57847077185));
#22948=CARTESIAN_POINT('Ctrl Pts',(-68.0754970824227,0.00347138491776708,
-101.570642253064));
#22949=CARTESIAN_POINT('Ctrl Pts',(-68.0784041665282,0.00321016784256067,
-101.562695470325));
#22950=CARTESIAN_POINT('Ctrl Pts',(-68.0815330051506,0.00292902493645311,
-101.554142501145));
#22951=CARTESIAN_POINT('Ctrl Pts',(-68.0847129375145,0.00266197584741215,
-101.545452989185));
#22952=CARTESIAN_POINT('Ctrl Pts',(-68.0879165455134,0.00241261000501636,
-101.536700792837));
#22953=CARTESIAN_POINT('Ctrl Pts',(-68.0915250570899,0.00213172684783878,
-101.526842407588));
#22954=CARTESIAN_POINT('Ctrl Pts',(-68.0951633311921,0.0018734474831218,
-101.516905259307));
#22955=CARTESIAN_POINT('Ctrl Pts',(-68.0987689579156,0.00164207254706628,
-101.507058343113));
#22956=CARTESIAN_POINT('Ctrl Pts',(-68.1055598239953,0.00120629915025051,
-101.488512582751));
#22957=CARTESIAN_POINT('Ctrl Pts',(-68.1122324839578,0.000869036017442551,
-101.47029331438));
#22958=CARTESIAN_POINT('Ctrl Pts',(-68.1182843604923,0.000628923333716003,
-101.453763491701));
#22959=CARTESIAN_POINT('Ctrl Pts',(-68.1213794941397,0.000506121613892526,
-101.44530958322));
#22960=CARTESIAN_POINT('Ctrl Pts',(-68.1243116528745,0.000407933319930232,
-101.43729923241));
#22961=CARTESIAN_POINT('Ctrl Pts',(-68.1270242533874,0.000329996143664024,
-101.429886130252));
#22962=CARTESIAN_POINT('Ctrl Pts',(-68.1294687572354,0.000259761796076702,
-101.423205693281));
#22963=CARTESIAN_POINT('Ctrl Pts',(-68.1317347258719,0.000205884902874958,
-101.41701091811));
#22964=CARTESIAN_POINT('Ctrl Pts',(-68.1337950754692,0.000164141575941579,
-101.411375522026));
#22965=CARTESIAN_POINT('Ctrl Pts',(-68.1357220174725,0.000125101128567872,
-101.406105017722));
#22966=CARTESIAN_POINT('Ctrl Pts',(-68.1374689566186,9.66253224390965E-5,
-101.401324211194));
#22967=CARTESIAN_POINT('Ctrl Pts',(-68.1390295368681,7.52229498877099E-5,
-101.397050537999));
#22968=CARTESIAN_POINT('Ctrl Pts',(-68.1404811145484,5.53154787336606E-5,
-101.393075370028));
#22969=CARTESIAN_POINT('Ctrl Pts',(-68.1417714173016,4.15083053098491E-5,
-101.389539080716));
#22970=CARTESIAN_POINT('Ctrl Pts',(-68.1429106739615,3.14122065048217E-5,
-101.386413974701));
#22971=CARTESIAN_POINT('Ctrl Pts',(-68.1440153840732,2.16222594001115E-5,
-101.383383633658));
#22972=CARTESIAN_POINT('Ctrl Pts',(-68.144977967085,1.53159278963511E-5,
-101.380740200471));
#22973=CARTESIAN_POINT('Ctrl Pts',(-68.1458238660413,1.09001335344416E-5,
-101.378414522321));
#22974=CARTESIAN_POINT('Ctrl Pts',(-68.1466475415775,6.60035072704163E-6,
-101.376149944285));
#22975=CARTESIAN_POINT('Ctrl Pts',(-68.1473604970042,4.09626589672126E-6,
-101.374186883115));
#22976=CARTESIAN_POINT('Ctrl Pts',(-68.1480031204067,2.49220895143232E-6,
-101.372415415303));
#22977=CARTESIAN_POINT('Ctrl Pts',(-68.1486256515069,9.38304547818374E-7,
-101.370699334311));
#22978=CARTESIAN_POINT('Ctrl Pts',(-68.1491821314358,2.32998681033309E-7,
-101.369163186818));
#22979=CARTESIAN_POINT('Ctrl Pts',(-68.1497262923671,4.68224196081835E-8,
-101.367660612916));
#22980=CARTESIAN_POINT('Ctrl Pts',(-68.1498177332246,1.55373419849379E-8,
-101.367408120246));
#22981=CARTESIAN_POINT('Ctrl Pts',(-68.1499088672424,5.55111512312578E-16,
-101.367156463661));
#22982=CARTESIAN_POINT('Ctrl Pts',(-68.15,5.55111512312578E-16,-101.366904810515));
#22983=CARTESIAN_POINT('',(-68.2564581294845,2.08166817117217E-16,-101.658452405258));
#22984=CARTESIAN_POINT('Ctrl Pts',(-67.9629492358567,0.0221748193627332,
-101.882759497799));
#22985=CARTESIAN_POINT('Ctrl Pts',(-67.6593813619428,0.0951765737395145,
-102.737815214467));
#22986=CARTESIAN_POINT('Ctrl Pts',(-67.3499999997967,0.389138386673958,
-103.711832874224));
#22987=CARTESIAN_POINT('Ctrl Pts',(-67.35,0.800000000395794,-104.521316838008));
#22988=CARTESIAN_POINT('Ctrl Pts',(-68.0878075034141,0.0149175388607178,
-101.92835242401));
#22989=CARTESIAN_POINT('Ctrl Pts',(-67.7813554129666,0.0668886409596893,
-102.783387485583));
#22990=CARTESIAN_POINT('Ctrl Pts',(-67.4526591694531,0.338541460012509,
-103.754441947976));
#22991=CARTESIAN_POINT('Ctrl Pts',(-67.4229730822988,0.743827073473449,
-104.557333470599));
#22992=CARTESIAN_POINT('Ctrl Pts',(-68.2126657709715,0.00766025835870252,
-101.973945350221));
#22993=CARTESIAN_POINT('Ctrl Pts',(-67.9033294639905,0.0386007081798643,
-102.8289597567));
#22994=CARTESIAN_POINT('Ctrl Pts',(-67.5553183391094,0.287944533351058,
-103.797051021729));
#22995=CARTESIAN_POINT('Ctrl Pts',(-67.4959461645976,0.687654146551103,
-104.593350103189));
#22996=CARTESIAN_POINT('Ctrl Pts',(-68.3375240385289,0.000402977856687192,
-102.019538276432));
#22997=CARTESIAN_POINT('Ctrl Pts',(-68.0253035150143,0.0103127754000391,
-102.874532027816));
#22998=CARTESIAN_POINT('Ctrl Pts',(-67.6579775087658,0.237347606689609,
-103.839660095481));
#22999=CARTESIAN_POINT('Ctrl Pts',(-67.5689192468964,0.631481219628758,
-104.629366735779));
#23000=CARTESIAN_POINT('',(-67.5689192468964,0.631481219628695,-104.629366735779));
#23001=CARTESIAN_POINT('Ctrl Pts',(-68.3375240385289,0.000402977856687192,
-102.019538276432));
#23002=CARTESIAN_POINT('Ctrl Pts',(-68.0253035150143,0.0103127754000391,
-102.874532027816));
#23003=CARTESIAN_POINT('Ctrl Pts',(-67.6579775087658,0.237347606689609,
-103.839660095481));
#23004=CARTESIAN_POINT('Ctrl Pts',(-67.5689192468964,0.631481219628758,
-104.629366735779));
#23005=CARTESIAN_POINT('',(-67.35,0.800000000220445,-104.521316838097));
#23006=CARTESIAN_POINT('',(-67.5689192468964,0.631481219628695,-104.629366735779));
#23007=CARTESIAN_POINT('Ctrl Pts',(-67.35,0.800000000395794,-104.521316838008));
#23008=CARTESIAN_POINT('Ctrl Pts',(-67.3499999997967,0.389138386673958,
-103.711832874224));
#23009=CARTESIAN_POINT('Ctrl Pts',(-67.6593813619428,0.0951765737395145,
-102.737815214467));
#23010=CARTESIAN_POINT('Ctrl Pts',(-67.9629492358567,0.0221748193627332,
-101.882759497799));
#23011=CARTESIAN_POINT('Origin',(-67.45,6.00000000000001,-101.95));
#23012=CARTESIAN_POINT('',(-67.55,3.00667409058086,-107.15));
#23013=CARTESIAN_POINT('',(-67.35,3.10645162089483,-106.976666666667));
#23014=CARTESIAN_POINT('',(-67.55,3.00667409058086,-107.15));
#23015=CARTESIAN_POINT('',(-67.35,0.97333333333333,-104.843548379105));
#23016=CARTESIAN_POINT('Origin',(-67.35,6.00000000000001,-101.95));
#23017=CARTESIAN_POINT('',(-67.55,0.800000000000001,-104.943325909419));
#23018=CARTESIAN_POINT('',(-67.35,0.97333333333333,-104.843548379105));
#23019=CARTESIAN_POINT('Origin',(-67.55,6.00000000000001,-101.95));
#23020=CARTESIAN_POINT('Ctrl Pts',(-67.35,0.80000000039573,-104.521316838008));
#23021=CARTESIAN_POINT('Ctrl Pts',(-67.35,0.856168534250959,-104.631980686636));
#23022=CARTESIAN_POINT('Ctrl Pts',(-67.35,0.913326151321769,-104.739304018183));
#23023=CARTESIAN_POINT('Ctrl Pts',(-67.35,0.97333333333333,-104.843548379105));
#23024=CARTESIAN_POINT('Ctrl Pts',(-67.4229730822988,0.743827073473387,
-104.557333470599));
#23025=CARTESIAN_POINT('Ctrl Pts',(-67.4189147231253,0.79923331718401,-104.667096072329));
#23026=CARTESIAN_POINT('Ctrl Pts',(-67.4166666666667,0.856146146238358,
-104.773601644526));
#23027=CARTESIAN_POINT('Ctrl Pts',(-67.4166666666667,0.915555555555552,
-104.876807555876));
#23028=CARTESIAN_POINT('Ctrl Pts',(-67.4959461645976,0.687654146551043,
-104.593350103189));
#23029=CARTESIAN_POINT('Ctrl Pts',(-67.4878294462506,0.742298100117062,
-104.702211458022));
#23030=CARTESIAN_POINT('Ctrl Pts',(-67.4833333333333,0.798966141154948,
-104.80789927087));
#23031=CARTESIAN_POINT('Ctrl Pts',(-67.4833333333333,0.857777777777775,
-104.910066732648));
#23032=CARTESIAN_POINT('Ctrl Pts',(-67.5689192468964,0.6314812196287,-104.629366735779));
#23033=CARTESIAN_POINT('Ctrl Pts',(-67.556744169376,0.685362883050113,-104.737326843716));
#23034=CARTESIAN_POINT('Ctrl Pts',(-67.55,0.741786136071537,-104.842196897214));
#23035=CARTESIAN_POINT('Ctrl Pts',(-67.55,0.799999999999996,-104.943325909419));
#23036=CARTESIAN_POINT('Ctrl Pts',(-67.35,0.97333333333333,-104.843548379105));
#23037=CARTESIAN_POINT('Ctrl Pts',(-67.35,0.913326151321769,-104.739304018183));
#23038=CARTESIAN_POINT('Ctrl Pts',(-67.35,0.856168534250959,-104.631980686636));
#23039=CARTESIAN_POINT('Ctrl Pts',(-67.35,0.80000000039573,-104.521316838008));
#23040=CARTESIAN_POINT('Ctrl Pts',(-67.5689192468964,0.6314812196287,-104.629366735779));
#23041=CARTESIAN_POINT('Ctrl Pts',(-67.556744169376,0.685362883050113,-104.737326843716));
#23042=CARTESIAN_POINT('Ctrl Pts',(-67.55,0.741786136071537,-104.842196897214));
#23043=CARTESIAN_POINT('Ctrl Pts',(-67.55,0.799999999999996,-104.943325909419));
#23044=CARTESIAN_POINT('Ctrl Pts',(-67.35,3.42868316199157,-107.149999999604));
#23045=CARTESIAN_POINT('Ctrl Pts',(-67.3499999999122,3.7782413927739,-107.327421746315));
#23046=CARTESIAN_POINT('Ctrl Pts',(-67.4083761721518,4.15716092828445,-107.487589107692));
#23047=CARTESIAN_POINT('Ctrl Pts',(-67.6167732367314,5.05523993056306,-107.780574427439));
#23048=CARTESIAN_POINT('Ctrl Pts',(-67.7904716797,5.58142525252587,-107.886348035845));
#23049=CARTESIAN_POINT('Ctrl Pts',(-67.9629497348173,6.06724190764723,-107.927825300627));
#23050=CARTESIAN_POINT('Ctrl Pts',(-67.4229730822988,3.39266652940126,-107.206172926527));
#23051=CARTESIAN_POINT('Ctrl Pts',(-67.4358232888358,3.73937765477556,-107.381196742291));
#23052=CARTESIAN_POINT('Ctrl Pts',(-67.5053957022727,4.11610756215676,-107.53590250564));
#23053=CARTESIAN_POINT('Ctrl Pts',(-67.7336142169646,5.0105732143284,-107.812221615036));
#23054=CARTESIAN_POINT('Ctrl Pts',(-67.9137670393935,5.53583525927463,-107.905551823189));
#23055=CARTESIAN_POINT('Ctrl Pts',(-68.0878080075958,6.02164898271821,-107.935082546577));
#23056=CARTESIAN_POINT('Ctrl Pts',(-67.4959461645976,3.35664989681094,-107.262345853449));
#23057=CARTESIAN_POINT('Ctrl Pts',(-67.5215538519502,3.70051482143448,-107.434941903931));
#23058=CARTESIAN_POINT('Ctrl Pts',(-67.6024177035411,4.07505262722886,-107.584215982616));
#23059=CARTESIAN_POINT('Ctrl Pts',(-67.8503982285565,4.96591111071775,-107.843862211275));
#23060=CARTESIAN_POINT('Ctrl Pts',(-68.0368334977355,5.49026758263733,-107.924762872196));
#23061=CARTESIAN_POINT('Ctrl Pts',(-68.2126662803743,5.97605605778919,-107.942339792527));
#23062=CARTESIAN_POINT('Ctrl Pts',(-67.5689192468964,3.32063326422062,-107.318518780371));
#23063=CARTESIAN_POINT('Ctrl Pts',(-67.6073771408738,3.66165108343613,-107.488716899907));
#23064=CARTESIAN_POINT('Ctrl Pts',(-67.699437233662,4.03399926110116,-107.632529380564));
#23065=CARTESIAN_POINT('Ctrl Pts',(-67.9672392087896,4.92124439448309,-107.875509398871));
#23066=CARTESIAN_POINT('Ctrl Pts',(-68.1601288574289,5.44467758938609,-107.943966659541));
#23067=CARTESIAN_POINT('Ctrl Pts',(-68.3375245531529,5.93046313286018,-107.949597038478));
#23068=CARTESIAN_POINT('',(-67.35,3.42868316190273,-107.14999999978));
#23069=CARTESIAN_POINT('Ctrl Pts',(-67.9629497348173,6.06724190764723,-107.927825300627));
#23070=CARTESIAN_POINT('Ctrl Pts',(-67.7904716797,5.58142525252587,-107.886348035845));
#23071=CARTESIAN_POINT('Ctrl Pts',(-67.6167732367314,5.05523993056306,-107.780574427439));
#23072=CARTESIAN_POINT('Ctrl Pts',(-67.4083761721518,4.15716092828445,-107.487589107692));
#23073=CARTESIAN_POINT('Ctrl Pts',(-67.3499999999122,3.7782413927739,-107.327421746315));
#23074=CARTESIAN_POINT('Ctrl Pts',(-67.35,3.42868316199157,-107.149999999604));
#23075=CARTESIAN_POINT('',(-67.5689192468964,3.32063326422074,-107.318518780371));
#23076=CARTESIAN_POINT('',(-67.35,3.42868316190273,-107.14999999978));
#23077=CARTESIAN_POINT('Ctrl Pts',(-67.5689192468964,3.32063326422062,-107.318518780371));
#23078=CARTESIAN_POINT('Ctrl Pts',(-67.6073771408738,3.66165108343613,-107.488716899907));
#23079=CARTESIAN_POINT('Ctrl Pts',(-67.699437233662,4.03399926110116,-107.632529380564));
#23080=CARTESIAN_POINT('Ctrl Pts',(-67.9672392087896,4.92124439448309,-107.875509398871));
#23081=CARTESIAN_POINT('Ctrl Pts',(-68.1601288574289,5.44467758938609,-107.943966659541));
#23082=CARTESIAN_POINT('Ctrl Pts',(-68.3375245531529,5.93046313286018,-107.949597038478));
#23083=CARTESIAN_POINT('Ctrl Pts',(-67.35,3.10645162089483,-106.976666666667));
#23084=CARTESIAN_POINT('Ctrl Pts',(-67.35,3.21069598181732,-107.036673848678));
#23085=CARTESIAN_POINT('Ctrl Pts',(-67.35,3.31801931336452,-107.093831465749));
#23086=CARTESIAN_POINT('Ctrl Pts',(-67.35,3.42868316199169,-107.149999999604));
#23087=CARTESIAN_POINT('Ctrl Pts',(-67.4166666666667,3.07319244412351,-107.034444444444));
#23088=CARTESIAN_POINT('Ctrl Pts',(-67.4166666666667,3.17639835547359,-107.093853853762));
#23089=CARTESIAN_POINT('Ctrl Pts',(-67.4189147231253,3.28290392767118,-107.150766682816));
#23090=CARTESIAN_POINT('Ctrl Pts',(-67.4229730822988,3.39266652940138,-107.206172926527));
#23091=CARTESIAN_POINT('Ctrl Pts',(-67.4833333333333,3.03993326735218,-107.092222222222));
#23092=CARTESIAN_POINT('Ctrl Pts',(-67.4833333333333,3.14210072912986,-107.151033858845));
#23093=CARTESIAN_POINT('Ctrl Pts',(-67.4878294462506,3.24778854197784,-107.207701899883));
#23094=CARTESIAN_POINT('Ctrl Pts',(-67.4959461645976,3.35664989681106,-107.262345853449));
#23095=CARTESIAN_POINT('Ctrl Pts',(-67.55,3.00667409058086,-107.15));
#23096=CARTESIAN_POINT('Ctrl Pts',(-67.55,3.10780310278613,-107.208213863928));
#23097=CARTESIAN_POINT('Ctrl Pts',(-67.556744169376,3.2126731562845,-107.26463711695));
#23098=CARTESIAN_POINT('Ctrl Pts',(-67.5689192468964,3.32063326422074,-107.318518780371));
#23099=CARTESIAN_POINT('Ctrl Pts',(-67.35,3.42868316199169,-107.149999999604));
#23100=CARTESIAN_POINT('Ctrl Pts',(-67.35,3.31801931336452,-107.093831465749));
#23101=CARTESIAN_POINT('Ctrl Pts',(-67.35,3.21069598181732,-107.036673848678));
#23102=CARTESIAN_POINT('Ctrl Pts',(-67.35,3.10645162089483,-106.976666666667));
#23103=CARTESIAN_POINT('Ctrl Pts',(-67.55,3.00667409058086,-107.15));
#23104=CARTESIAN_POINT('Ctrl Pts',(-67.55,3.10780310278613,-107.208213863928));
#23105=CARTESIAN_POINT('Ctrl Pts',(-67.556744169376,3.2126731562845,-107.26463711695));
#23106=CARTESIAN_POINT('Ctrl Pts',(-67.5689192468964,3.32063326422074,-107.318518780371));
#23107=CARTESIAN_POINT('Origin',(-68.15,92.25,-107.15));
#23108=CARTESIAN_POINT('',(-68.15,121.,-107.95));
#23109=CARTESIAN_POINT('',(-68.15,92.25,-107.95));
#23110=CARTESIAN_POINT('',(-67.35,123.993325909419,-107.15));
#23111=CARTESIAN_POINT('Ctrl Pts',(-68.15,121.,-107.95));
#23112=CARTESIAN_POINT('Ctrl Pts',(-67.9725091568851,121.486078692623,-107.95));
#23113=CARTESIAN_POINT('Ctrl Pts',(-67.7780133341431,122.014025751789,-107.887608349819));
#23114=CARTESIAN_POINT('Ctrl Pts',(-67.4681119224052,123.043713064318,-107.61628036626));
#23115=CARTESIAN_POINT('Ctrl Pts',(-67.35,123.544851663295,-107.408159534737));
#23116=CARTESIAN_POINT('Ctrl Pts',(-67.35,123.993325909419,-107.15));
#23117=CARTESIAN_POINT('',(-67.35,92.25,-107.15));
#23118=CARTESIAN_POINT('Origin',(-67.35,121.,-107.95));
#23119=CARTESIAN_POINT('',(-71.099583741031,6.,-107.95));
#23120=CARTESIAN_POINT('',(-67.35,6.,-107.95));
#23121=CARTESIAN_POINT('',(-71.3125,6.58309518948457,-107.95));
#23122=CARTESIAN_POINT('',(-71.2060418705155,6.29154759474228,-107.95));
#23123=CARTESIAN_POINT('',(-71.3125,121.,-107.95));
#23124=CARTESIAN_POINT('',(-71.3125,92.25,-107.95));
#23125=CARTESIAN_POINT('',(-67.35,121.,-107.95));
#23126=CARTESIAN_POINT('Origin',(-67.35,6.00000000000001,-101.95));
#23127=CARTESIAN_POINT('',(-71.099583741031,0.,-101.95));
#23128=CARTESIAN_POINT('',(-67.35,0.,-101.95));
#23129=CARTESIAN_POINT('',(-71.1249754475493,0.000402961545106217,-102.019536869093));
#23130=CARTESIAN_POINT('Ctrl Pts',(-71.1249754475493,0.000402961545105995,
-102.019536869093));
#23131=CARTESIAN_POINT('Ctrl Pts',(-71.124851587799,0.00039903034867228,
-102.019197687954));
#23132=CARTESIAN_POINT('Ctrl Pts',(-71.1247261194153,0.000395071000824783,
-102.01885410149));
#23133=CARTESIAN_POINT('Ctrl Pts',(-71.1245663846202,0.000390082845616924,
-102.018416679127));
#23134=CARTESIAN_POINT('Ctrl Pts',(-71.1243992161203,0.000384862552676827,
-102.017958900093));
#23135=CARTESIAN_POINT('Ctrl Pts',(-71.124194657536,0.00037851896831914,
-102.017398731222));
#23136=CARTESIAN_POINT('Ctrl Pts',(-71.1239352655514,0.000370623381937385,
-102.016688403951));
#23137=CARTESIAN_POINT('Ctrl Pts',(-71.1236418508271,0.000361692183446622,
-102.015884907726));
#23138=CARTESIAN_POINT('Ctrl Pts',(-71.123278284165,0.000350777273635938,
-102.014889304042));
#23139=CARTESIAN_POINT('Ctrl Pts',(-71.1228435347465,0.000338137262748894,
-102.013698766206));
#23140=CARTESIAN_POINT('Ctrl Pts',(-71.1223678613857,0.000324307419154685,
-102.012396160361));
#23141=CARTESIAN_POINT('Ctrl Pts',(-71.1218074193177,0.000308441358892688,
-102.010861414961));
#23142=CARTESIAN_POINT('Ctrl Pts',(-71.1211844502614,0.000291620849225183,
-102.009155432109));
#23143=CARTESIAN_POINT('Ctrl Pts',(-71.1202527752878,0.000266465108755621,
-102.006604066976));
#23144=CARTESIAN_POINT('Ctrl Pts',(-71.1191829299107,0.000239334834657964,
-102.003674304497));
#23145=CARTESIAN_POINT('Ctrl Pts',(-71.1180892999079,0.000214037091799568,
-102.000679377361));
#23146=CARTESIAN_POINT('Ctrl Pts',(-71.1173517759251,0.00019697675876076,
-101.99865965352));
#23147=CARTESIAN_POINT('Ctrl Pts',(-71.1166045457774,0.00018073635052839,
-101.996613335964));
#23148=CARTESIAN_POINT('Ctrl Pts',(-71.1158742950379,0.000165866021002437,
-101.994613504015));
#23149=CARTESIAN_POINT('Ctrl Pts',(-71.1152379645436,0.00015290821948918,
-101.992870877841));
#23150=CARTESIAN_POINT('Ctrl Pts',(-71.1146147686253,0.000140979678841012,
-101.991164211349));
#23151=CARTESIAN_POINT('Ctrl Pts',(-71.1140085827462,0.000130049362750739,
-101.989504119281));
#23152=CARTESIAN_POINT('Ctrl Pts',(-71.1134416133361,0.000119826170360816,
-101.98795142488));
#23153=CARTESIAN_POINT('Ctrl Pts',(-71.1128897131664,0.000110468349252261,
-101.986439991042));
#23154=CARTESIAN_POINT('Ctrl Pts',(-71.1123401816121,0.00010170560401157,
-101.984935038344));
#23155=CARTESIAN_POINT('Ctrl Pts',(-71.1117897479163,9.29284733604459E-5,
-101.983427615032));
#23156=CARTESIAN_POINT('Ctrl Pts',(-71.1112385933679,8.46980842703503E-5,
-101.98191821223));
#23157=CARTESIAN_POINT('Ctrl Pts',(-71.1106726308321,7.68530591930272E-5,
-101.980368253225));
#23158=CARTESIAN_POINT('Ctrl Pts',(-71.1100599017399,6.83597848340904E-5,
-101.978690218171));
#23159=CARTESIAN_POINT('Ctrl Pts',(-71.1094299982868,6.03342636038971E-5,
-101.976965145765));
#23160=CARTESIAN_POINT('Ctrl Pts',(-71.1087859004829,5.29252693262094E-5,
-101.975201198996));
#23161=CARTESIAN_POINT('Ctrl Pts',(-71.1080330497704,4.42653009376351E-5,
-101.973139418046));
#23162=CARTESIAN_POINT('Ctrl Pts',(-71.1072611035879,3.64757776301905E-5,
-101.971025339841));
#23163=CARTESIAN_POINT('Ctrl Pts',(-71.1064989308872,2.98874829738338E-5,
-101.968938027944));
#23164=CARTESIAN_POINT('Ctrl Pts',(-71.1055840060273,2.19787838566663E-5,
-101.966432383826));
#23165=CARTESIAN_POINT('Ctrl Pts',(-71.1046847841119,1.58466565800604E-5,
-101.963969744833));
#23166=CARTESIAN_POINT('Ctrl Pts',(-71.1038687722318,1.14758458700237E-5,
-101.961734991212));
#23167=CARTESIAN_POINT('Ctrl Pts',(-71.1032398031926,8.10689416688974E-6,
-101.960012478498));
#23168=CARTESIAN_POINT('Ctrl Pts',(-71.102661057005,5.75949607614505E-6,
-101.958427509908));
#23169=CARTESIAN_POINT('Ctrl Pts',(-71.1021565448688,4.1369944820957E-6,
-101.957045843929));
#23170=CARTESIAN_POINT('Ctrl Pts',(-71.1016982611712,2.66316268176917E-6,
-101.95579077998));
#23171=CARTESIAN_POINT('Ctrl Pts',(-71.1013015498054,1.77620578348578E-6,
-101.954704342338));
#23172=CARTESIAN_POINT('Ctrl Pts',(-71.1009716248581,1.20384665613926E-6,
-101.953800810232));
#23173=CARTESIAN_POINT('Ctrl Pts',(-71.1006620429046,6.66778882898464E-7,
-101.952952989427));
#23174=CARTESIAN_POINT('Ctrl Pts',(-71.1004114665276,4.02530372668449E-7,
-101.952266765024));
#23175=CARTESIAN_POINT('Ctrl Pts',(-71.1002088602548,2.44220883516277E-7,
-101.951711914293));
#23176=CARTESIAN_POINT('Ctrl Pts',(-71.1000192697177,9.60814371089195E-8,
-101.951192708018));
#23177=CARTESIAN_POINT('Ctrl Pts',(-71.099871769579,4.12488911489826E-8,
-101.950788772905));
#23178=CARTESIAN_POINT('Ctrl Pts',(-71.0997415471677,1.55631951770374E-8,
-101.950432155465));
#23179=CARTESIAN_POINT('Ctrl Pts',(-71.0996870475923,4.8134362897241E-9,
-101.950282906969));
#23180=CARTESIAN_POINT('Ctrl Pts',(-71.0996353689583,0.,-101.950141384051));
#23181=CARTESIAN_POINT('Ctrl Pts',(-71.099583741031,0.,-101.95));
#23182=CARTESIAN_POINT('',(-71.8935807531036,0.631481219628703,-104.629366735779));
#23183=CARTESIAN_POINT('Ctrl Pts',(-71.8935807531036,0.63148121962876,-104.629366735779));
#23184=CARTESIAN_POINT('Ctrl Pts',(-71.8045224423712,0.237347390442852,
-103.839659662198));
#23185=CARTESIAN_POINT('Ctrl Pts',(-71.4371961129181,0.0103125630353027,
-102.874531011475));
#23186=CARTESIAN_POINT('Ctrl Pts',(-71.1249754475488,0.000402961545087344,
-102.019536869091));
#23187=CARTESIAN_POINT('',(-71.9125,0.800000000000001,-104.943325909419));
#23188=CARTESIAN_POINT('Ctrl Pts',(-71.9125,0.800000000000002,-104.943325909419));
#23189=CARTESIAN_POINT('Ctrl Pts',(-71.9125,0.741786136071551,-104.842196897214));
#23190=CARTESIAN_POINT('Ctrl Pts',(-71.905755830624,0.685362883050117,-104.737326843716));
#23191=CARTESIAN_POINT('Ctrl Pts',(-71.8935807531036,0.631481219628707,
-104.629366735779));
#23192=CARTESIAN_POINT('',(-71.9125,3.00667409058086,-107.15));
#23193=CARTESIAN_POINT('Origin',(-71.9125,6.00000000000001,-101.95));
#23194=CARTESIAN_POINT('',(-71.8935807531036,3.32063326422075,-107.318518780371));
#23195=CARTESIAN_POINT('Ctrl Pts',(-71.8935807531036,3.32063326422075,-107.318518780371));
#23196=CARTESIAN_POINT('Ctrl Pts',(-71.905755830624,3.2126731562845,-107.26463711695));
#23197=CARTESIAN_POINT('Ctrl Pts',(-71.9125,3.10780310278613,-107.208213863928));
#23198=CARTESIAN_POINT('Ctrl Pts',(-71.9125,3.00667409058086,-107.15));
#23199=CARTESIAN_POINT('',(-71.124975960152,5.93046172723723,-107.949597022186));
#23200=CARTESIAN_POINT('Ctrl Pts',(-71.124975960152,5.93046172723723,-107.949597022186));
#23201=CARTESIAN_POINT('Ctrl Pts',(-71.4371989024855,5.0754613003514,-107.939687147793));
#23202=CARTESIAN_POINT('Ctrl Pts',(-71.8045224912342,4.11033990451893,-107.71265239331));
#23203=CARTESIAN_POINT('Ctrl Pts',(-71.8935807531036,3.32063326422062,-107.318518780371));
#23204=CARTESIAN_POINT('Ctrl Pts',(-71.099583741031,6.,-107.95));
#23205=CARTESIAN_POINT('Ctrl Pts',(-71.0997076101999,5.99966078194888,-107.95));
#23206=CARTESIAN_POINT('Ctrl Pts',(-71.0998330879657,5.99931715853558,-107.949999977092));
#23207=CARTESIAN_POINT('Ctrl Pts',(-71.0999928315222,5.99887969296171,-107.949999895409));
#23208=CARTESIAN_POINT('Ctrl Pts',(-71.1001600092056,5.99842186866603,-107.949999809925));
#23209=CARTESIAN_POINT('Ctrl Pts',(-71.1003645763045,5.99786164766841,-107.949999661008));
#23210=CARTESIAN_POINT('Ctrl Pts',(-71.100623975913,5.99715125904428,-107.949999323723));
#23211=CARTESIAN_POINT('Ctrl Pts',(-71.1009173990571,5.99634769397783,-107.949998942198));
#23212=CARTESIAN_POINT('Ctrl Pts',(-71.1012809729018,5.99535200993297,-107.949998317815));
#23213=CARTESIAN_POINT('Ctrl Pts',(-71.1017157284528,5.99416138284706,-107.949997159212));
#23214=CARTESIAN_POINT('Ctrl Pts',(-71.1021914073829,5.99285868247456,-107.94999589155));
#23215=CARTESIAN_POINT('Ctrl Pts',(-71.1027518533654,5.99132383326823,-107.94999396957));
#23216=CARTESIAN_POINT('Ctrl Pts',(-71.1033748255994,5.98961774499851,-107.949991017392));
#23217=CARTESIAN_POINT('Ctrl Pts',(-71.1043065151119,5.98706619540861,-107.949986602245));
#23218=CARTESIAN_POINT('Ctrl Pts',(-71.1053763764072,5.9841362381271,-107.949979775947));
#23219=CARTESIAN_POINT('Ctrl Pts',(-71.106470023737,5.98114113876118,-107.949970361873));
#23220=CARTESIAN_POINT('Ctrl Pts',(-71.1072075567092,5.97912130615377,-107.949964013218));
#23221=CARTESIAN_POINT('Ctrl Pts',(-71.1079547963995,5.9770748900843,-107.949956536432));
#23222=CARTESIAN_POINT('Ctrl Pts',(-71.1086850574233,5.97507497391498,-107.949948228366));
#23223=CARTESIAN_POINT('Ctrl Pts',(-71.1093213960554,5.97333227660838,-107.949940988841));
#23224=CARTESIAN_POINT('Ctrl Pts',(-71.1099446007125,5.97162554958123,-107.949933136853));
#23225=CARTESIAN_POINT('Ctrl Pts',(-71.1105507958981,5.96996540809479,-107.94992482647));
#23226=CARTESIAN_POINT('Ctrl Pts',(-71.1111177706135,5.9684126767813,-107.949917053764));
#23227=CARTESIAN_POINT('Ctrl Pts',(-71.1116696767866,5.96690121509207,-107.949908893929));
#23228=CARTESIAN_POINT('Ctrl Pts',(-71.112219214484,5.96539624482729,-107.949900214181));
#23229=CARTESIAN_POINT('Ctrl Pts',(-71.112769657144,5.96388879622165,-107.949891520139));
#23230=CARTESIAN_POINT('Ctrl Pts',(-71.1133208207184,5.96237937864895,-107.949882256457));
#23231=CARTESIAN_POINT('Ctrl Pts',(-71.1138867930719,5.96082941367587,-107.949872137401));
#23232=CARTESIAN_POINT('Ctrl Pts',(-71.1144995294067,5.95915138143476,-107.94986118225));
#23233=CARTESIAN_POINT('Ctrl Pts',(-71.1151294408272,5.95742632285292,-107.949849214239));
#23234=CARTESIAN_POINT('Ctrl Pts',(-71.1157735476843,5.95566239958307,-107.949836179196));
#23235=CARTESIAN_POINT('Ctrl Pts',(-71.1165264025987,5.95360066357222,-107.949820943375));
#23236=CARTESIAN_POINT('Ctrl Pts',(-71.117298354139,5.95148664466337,-107.949804231078));
#23237=CARTESIAN_POINT('Ctrl Pts',(-71.1180605342385,5.94939939913612,-107.949786627805));
#23238=CARTESIAN_POINT('Ctrl Pts',(-71.1189754957585,5.94689375861683,-107.949765495901));
#23239=CARTESIAN_POINT('Ctrl Pts',(-71.1198747564399,5.94443113581304,-107.949743085817));
#23240=CARTESIAN_POINT('Ctrl Pts',(-71.1206908036366,5.94219640766141,-107.949721555598));
#23241=CARTESIAN_POINT('Ctrl Pts',(-71.1213197924908,5.94047393486156,-107.949704960642));
#23242=CARTESIAN_POINT('Ctrl Pts',(-71.1218985575461,5.93888900822262,-107.949688938252));
#23243=CARTESIAN_POINT('Ctrl Pts',(-71.1224030859461,5.93750738102305,-107.949674547221));
#23244=CARTESIAN_POINT('Ctrl Pts',(-71.1228613835834,5.93625235458417,-107.949661474864));
#23245=CARTESIAN_POINT('Ctrl Pts',(-71.123258106951,5.93516595105505,-107.949649769988));
#23246=CARTESIAN_POINT('Ctrl Pts',(-71.1235880409681,5.93426244786692,-107.949639870379));
#23247=CARTESIAN_POINT('Ctrl Pts',(-71.1238976311937,5.93341465484948,-107.949630581182));
#23248=CARTESIAN_POINT('Ctrl Pts',(-71.1241482133456,5.93272845333488,-107.949622892056));
#23249=CARTESIAN_POINT('Ctrl Pts',(-71.1243508223328,5.93217362299574,-107.949616619633));
#23250=CARTESIAN_POINT('Ctrl Pts',(-71.1245404151432,5.93165443653311,-107.949610750169));
#23251=CARTESIAN_POINT('Ctrl Pts',(-71.1246879149935,5.93125051870808,-107.949606123405));
#23252=CARTESIAN_POINT('Ctrl Pts',(-71.1248181342775,5.93089392231776,-107.94960201597));
#23253=CARTESIAN_POINT('Ctrl Pts',(-71.1248726413951,5.93074465839334,-107.949600296682));
#23254=CARTESIAN_POINT('Ctrl Pts',(-71.124924326144,5.93060312331329,-107.949598661036));
#23255=CARTESIAN_POINT('Ctrl Pts',(-71.124975960152,5.93046172723723,-107.949597022186));
#23256=CARTESIAN_POINT('Ctrl Pts',(-67.9629497353525,0.0221746992445629,
38.3827580908684));
#23257=CARTESIAN_POINT('Ctrl Pts',(-67.9731885882307,0.0197124752224134,
38.3539184501918));
#23258=CARTESIAN_POINT('Ctrl Pts',(-68.0649766144896,-0.000362008710208082,
38.0974285502451));
#23259=CARTESIAN_POINT('Ctrl Pts',(-68.142152319925,6.41557585660516E-16,
37.8885753209566));
#23260=CARTESIAN_POINT('Ctrl Pts',(-68.15,5.55111512312588E-16,37.8669048105155));
#23261=CARTESIAN_POINT('Ctrl Pts',(-68.0878080077735,0.014917453342971,
38.4283510167903));
#23262=CARTESIAN_POINT('Ctrl Pts',(-68.0951549181673,0.0138762587036523,
38.4077957764774));
#23263=CARTESIAN_POINT('Ctrl Pts',(-68.1598892716053,-0.00240660968547253,
38.2259097718945));
#23264=CARTESIAN_POINT('Ctrl Pts',(-68.2153859993257,1.16858226445236E-15,
38.0766871386273));
#23265=CARTESIAN_POINT('Ctrl Pts',(-68.220972086323,1.11022302462517E-15,
38.061269873677));
#23266=CARTESIAN_POINT('Ctrl Pts',(-68.2126662801947,0.00766020744137906,
38.4739439427121));
#23267=CARTESIAN_POINT('Ctrl Pts',(-68.2170579360371,0.00742672694733014,
38.4617488613535));
#23268=CARTESIAN_POINT('Ctrl Pts',(-68.2567225636689,0.00233198877221449,
38.3525319855683));
#23269=CARTESIAN_POINT('Ctrl Pts',(-68.2886196787263,1.69564431891977E-15,
38.264798956298));
#23270=CARTESIAN_POINT('Ctrl Pts',(-68.291944172646,1.66533453693774E-15,
38.2556349368385));
#23271=CARTESIAN_POINT('Ctrl Pts',(-68.3375245526157,0.000402961539787139,
38.5195368686339));
#23272=CARTESIAN_POINT('Ctrl Pts',(-68.3389416666765,0.000357983621347725,
38.5156562022828));
#23273=CARTESIAN_POINT('Ctrl Pts',(-68.3515732880386,-7.64792169922838E-6,
38.4810647510841));
#23274=CARTESIAN_POINT('Ctrl Pts',(-68.3618533581269,2.22267096799525E-15,
38.4529107739687));
#23275=CARTESIAN_POINT('Ctrl Pts',(-68.3629162589689,2.22044604925032E-15,
38.45));
#23276=CARTESIAN_POINT('',(-68.15,5.55111512312578E-16,37.8669048105155));
#23277=CARTESIAN_POINT('',(-67.9629497353525,0.0221746992445629,38.3827580908684));
#23278=CARTESIAN_POINT('Ctrl Pts',(-68.15,5.55111512312578E-16,37.8669048105155));
#23279=CARTESIAN_POINT('Ctrl Pts',(-68.1494585269693,5.61123070571811E-16,
37.8684000290838));
#23280=CARTESIAN_POINT('Ctrl Pts',(-68.1489155383042,5.09286916023732E-7,
37.8698993845373));
#23281=CARTESIAN_POINT('Ctrl Pts',(-68.1483145418308,1.77548274582495E-6,
37.8715567710143));
#23282=CARTESIAN_POINT('Ctrl Pts',(-68.1476856008852,3.10055275502112E-6,
37.8732912208225));
#23283=CARTESIAN_POINT('Ctrl Pts',(-68.1469931402788,5.24993589625362E-6,
37.8751987160141));
#23284=CARTESIAN_POINT('Ctrl Pts',(-68.14619231509,9.06159155444897E-6,
37.8774013289947));
#23285=CARTESIAN_POINT('Ctrl Pts',(-68.1453619255287,1.30139635753023E-5,
37.8796852566885));
#23286=CARTESIAN_POINT('Ctrl Pts',(-68.1444150906901,1.87480333346877E-5,
37.8822863058685));
#23287=CARTESIAN_POINT('Ctrl Pts',(-68.1433221007964,2.78719466376698E-5,
37.8852852462417));
#23288=CARTESIAN_POINT('Ctrl Pts',(-68.1421797918381,3.74075589610416E-5,
37.8884195080249));
#23289=CARTESIAN_POINT('Ctrl Pts',(-68.1408779239497,5.06497820057028E-5,
37.8919881465915));
#23290=CARTESIAN_POINT('Ctrl Pts',(-68.1394032022783,7.01856549885083E-5,
37.8960271871082));
#23291=CARTESIAN_POINT('Ctrl Pts',(-68.1378429803325,9.08541637308448E-5,
37.9003003999972));
#23292=CARTESIAN_POINT('Ctrl Pts',(-68.1360893895847,0.000118592482698504,
37.9050998368976));
#23293=CARTESIAN_POINT('Ctrl Pts',(-68.1341478197916,0.000157072680741943,
37.910410677669));
#23294=CARTESIAN_POINT('Ctrl Pts',(-68.1320491213154,0.00019866703047275,
37.9161513177811));
#23295=CARTESIAN_POINT('Ctrl Pts',(-68.1297309455157,0.000252874501729824,
37.9224890449922));
#23296=CARTESIAN_POINT('Ctrl Pts',(-68.1272221199459,0.000324335633352324,
37.929345386396));
#23297=CARTESIAN_POINT('Ctrl Pts',(-68.1243771917707,0.000405370277300168,
37.9371202588592));
#23298=CARTESIAN_POINT('Ctrl Pts',(-68.1212874002126,0.000508732092038107,
37.9455612108248));
#23299=CARTESIAN_POINT('Ctrl Pts',(-68.1180188001475,0.000639503818214204,
37.954488825319));
#23300=CARTESIAN_POINT('Ctrl Pts',(-68.1129443831169,0.000842523539561197,
37.9683487158313));
#23301=CARTESIAN_POINT('Ctrl Pts',(-68.1074407997524,0.00111288779766146,
37.9833766395574));
#23302=CARTESIAN_POINT('Ctrl Pts',(-68.1018027353767,0.00145318003085737,
37.9987733555495));
#23303=CARTESIAN_POINT('Ctrl Pts',(-68.0982065898685,0.00167022976713585,
38.0085938945441));
#23304=CARTESIAN_POINT('Ctrl Pts',(-68.0945567832225,0.00191520573025482,
38.0185616386996));
#23305=CARTESIAN_POINT('Ctrl Pts',(-68.0909213110562,0.00218441447119044,
38.0284923792874));
#23306=CARTESIAN_POINT('Ctrl Pts',(-68.0875130559002,0.00243679766581759,
38.0378024485886));
#23307=CARTESIAN_POINT('Ctrl Pts',(-68.0841178992979,0.00271033441022534,
38.0470786218232));
#23308=CARTESIAN_POINT('Ctrl Pts',(-68.0807745892903,0.00300072615336044,
38.0562162719615));
#23309=CARTESIAN_POINT('Ctrl Pts',(-68.0778535622437,0.00325443942968668,
38.0641997742796));
#23310=CARTESIAN_POINT('Ctrl Pts',(-68.0749721105665,0.00352092683955299,
38.0720775254654));
#23311=CARTESIAN_POINT('Ctrl Pts',(-68.072139890947,0.00379788783359269,
38.0798240881857));
#23312=CARTESIAN_POINT('Ctrl Pts',(-68.0694783416282,0.00405815908513241,
38.0871038409948));
#23313=CARTESIAN_POINT('Ctrl Pts',(-68.0668603494036,0.00432761452089939,
38.094267506083));
#23314=CARTESIAN_POINT('Ctrl Pts',(-68.064277898257,0.00460593334325243,
38.1013380936256));
#23315=CARTESIAN_POINT('Ctrl Pts',(-68.061799078346,0.00487308350380365,
38.1081249454139));
#23316=CARTESIAN_POINT('Ctrl Pts',(-68.059353085522,0.00514834350309127,
38.1148258004088));
#23317=CARTESIAN_POINT('Ctrl Pts',(-68.0569163964528,0.00543380215951972,
38.1215064572704));
#23318=CARTESIAN_POINT('Ctrl Pts',(-68.0544290762057,0.00572519226950153,
38.1283259293509));
#23319=CARTESIAN_POINT('Ctrl Pts',(-68.0519486572191,0.00602751459370135,
38.135132075711));
#23320=CARTESIAN_POINT('Ctrl Pts',(-68.0494441195864,0.00634483879065095,
38.1420116774559));
#23321=CARTESIAN_POINT('Ctrl Pts',(-68.04685973585,0.00667227946593975,
38.1491106048705));
#23322=CARTESIAN_POINT('Ctrl Pts',(-68.0442497456397,0.00701574199235293,
38.1562875546711));
#23323=CARTESIAN_POINT('Ctrl Pts',(-68.0416005051211,0.00737805385543411,
38.1635814236488));
#23324=CARTESIAN_POINT('Ctrl Pts',(-68.0388040401881,0.00776050022555862,
38.1712806297719));
#23325=CARTESIAN_POINT('Ctrl Pts',(-68.0359639630212,0.00816399945284095,
38.1791097962615));
#23326=CARTESIAN_POINT('Ctrl Pts',(-68.0330849699915,0.00858931283554232,
38.1870570968145));
#23327=CARTESIAN_POINT('Ctrl Pts',(-68.0299863526566,0.00904707129720536,
38.1956106580789));
#23328=CARTESIAN_POINT('Ctrl Pts',(-68.0268428324837,0.00953016358578083,
38.2043006122038));
#23329=CARTESIAN_POINT('Ctrl Pts',(-68.02368140321,0.0100356893472873,38.213053049198));
#23330=CARTESIAN_POINT('Ctrl Pts',(-68.0201202624502,0.0106051306469534,
38.2229120899764));
#23331=CARTESIAN_POINT('Ctrl Pts',(-68.0165367020469,0.011203134184015,
38.2328496433373));
#23332=CARTESIAN_POINT('Ctrl Pts',(-68.0129916108277,0.0118193726711993,
38.2426965899744));
#23333=CARTESIAN_POINT('Ctrl Pts',(-68.0063167143977,0.0129796610315748,
38.2612369729688));
#23334=CARTESIAN_POINT('Ctrl Pts',(-67.9997811752937,0.0142069876584006,
38.2794496998821));
#23335=CARTESIAN_POINT('Ctrl Pts',(-67.993867728542,0.0153837155594101,
38.295972224156));
#23336=CARTESIAN_POINT('Ctrl Pts',(-67.9908424151136,0.0159857283735882,
38.3044251310064));
#23337=CARTESIAN_POINT('Ctrl Pts',(-67.9879803331532,0.0165735929941208,
38.3124339979299));
#23338=CARTESIAN_POINT('Ctrl Pts',(-67.9853349522781,0.0171300094787392,
38.3198450639127));
#23339=CARTESIAN_POINT('Ctrl Pts',(-67.9829511074834,0.0176314157424178,
38.3265234334561));
#23340=CARTESIAN_POINT('Ctrl Pts',(-67.9807434377889,0.0181071459725225,
38.3327157261395));
#23341=CARTESIAN_POINT('Ctrl Pts',(-67.9787370295873,0.0185468696297888,
38.3383482354825));
#23342=CARTESIAN_POINT('Ctrl Pts',(-67.9768605599421,0.0189581160025026,
38.3436159735227));
#23343=CARTESIAN_POINT('Ctrl Pts',(-67.9751602612767,0.0193377871914143,
38.3483936722831));
#23344=CARTESIAN_POINT('Ctrl Pts',(-67.9736414104918,0.0196810601384272,
38.3526639575534));
#23345=CARTESIAN_POINT('Ctrl Pts',(-67.9722286448025,0.02000035696892,38.3566359820428));
#23346=CARTESIAN_POINT('Ctrl Pts',(-67.9709729001376,0.0202881343017986,
38.3601688836916));
#23347=CARTESIAN_POINT('Ctrl Pts',(-67.9698637173153,0.02054447230098,38.3632904546014));
#23348=CARTESIAN_POINT('Ctrl Pts',(-67.9687881743821,0.0207930359444191,
38.3663173528415));
#23349=CARTESIAN_POINT('Ctrl Pts',(-67.9678505360297,0.0210120088053539,
38.3689572081709));
#23350=CARTESIAN_POINT('Ctrl Pts',(-67.9670258490686,0.021205765242865,
38.3712793095085));
#23351=CARTESIAN_POINT('Ctrl Pts',(-67.9662228312024,0.0213944306254464,
38.3735403963807));
#23352=CARTESIAN_POINT('Ctrl Pts',(-67.9655269913847,0.0215591701240771,
38.3754999694087));
#23353=CARTESIAN_POINT('Ctrl Pts',(-67.9648991165362,0.0217084974503975,
38.3772681263158));
#23354=CARTESIAN_POINT('Ctrl Pts',(-67.9642908652096,0.0218531577191369,
38.378981021468));
#23355=CARTESIAN_POINT('Ctrl Pts',(-67.9637464446629,0.0219833465228433,
38.3805141447143));
#23356=CARTESIAN_POINT('Ctrl Pts',(-67.9632138930181,0.0221112224498099,
38.3820140692215));
#23357=CARTESIAN_POINT('Ctrl Pts',(-67.9631256471495,0.0221324119858056,
38.3822626125173));
#23358=CARTESIAN_POINT('Ctrl Pts',(-67.9630376888859,0.0221535483104188,
38.3825103533209));
#23359=CARTESIAN_POINT('Ctrl Pts',(-67.9629497353525,0.0221746992445633,
38.3827580908684));
#23360=CARTESIAN_POINT('',(-68.3375245526157,0.000402961539787139,38.5195368686339));
#23361=CARTESIAN_POINT('Ctrl Pts',(-68.3375245526157,0.000402961539787139,
38.5195368686339));
#23362=CARTESIAN_POINT('Ctrl Pts',(-68.2126662801947,0.00766020744137906,
38.4739439427121));
#23363=CARTESIAN_POINT('Ctrl Pts',(-68.0878080077735,0.014917453342971,
38.4283510167903));
#23364=CARTESIAN_POINT('Ctrl Pts',(-67.9629497353525,0.0221746992445629,
38.3827580908684));
#23365=CARTESIAN_POINT('',(-68.3629162589689,2.22044604925031E-15,38.45));
#23366=CARTESIAN_POINT('Ctrl Pts',(-68.3375245526157,0.000402961539786695,
38.5195368686339));
#23367=CARTESIAN_POINT('Ctrl Pts',(-68.3376484123646,0.000399030343394364,
38.519197687496));
#23368=CARTESIAN_POINT('Ctrl Pts',(-68.3377738807469,0.000395070995587234,
38.5188541010336));
#23369=CARTESIAN_POINT('Ctrl Pts',(-68.3379336155403,0.000390082840428185,
38.5184166786719));
#23370=CARTESIAN_POINT('Ctrl Pts',(-68.3381007840383,0.00038486254753915,
38.5179588996392));
#23371=CARTESIAN_POINT('Ctrl Pts',(-68.3383053426202,0.000378518963241221,
38.5173987307702));
#23372=CARTESIAN_POINT('Ctrl Pts',(-68.338564734602,0.000370623376931611,
38.5166884035007));
#23373=CARTESIAN_POINT('Ctrl Pts',(-68.3388581493232,0.000361692178520524,
38.5158849072773));
#23374=CARTESIAN_POINT('Ctrl Pts',(-68.3392217159815,0.000350777268805274,
38.514889303595));
#23375=CARTESIAN_POINT('Ctrl Pts',(-68.3396564653955,0.000338137258031779,
38.5136987657616));
#23376=CARTESIAN_POINT('Ctrl Pts',(-68.3401321387519,0.000324307414550922,
38.5123961599182));
#23377=CARTESIAN_POINT('Ctrl Pts',(-68.3406925808146,0.000308441354420271,
38.5108614145199));
#23378=CARTESIAN_POINT('Ctrl Pts',(-68.3413155498654,0.000291620844902418,
38.5091554316702));
#23379=CARTESIAN_POINT('Ctrl Pts',(-68.3422472248276,0.000266465104742255,
38.5066040665502));
#23380=CARTESIAN_POINT('Ctrl Pts',(-68.3433170701914,0.000239334831008019,
38.5036743040879));
#23381=CARTESIAN_POINT('Ctrl Pts',(-68.3444107001817,0.000214037088507091,
38.5006793769712));
#23382=CARTESIAN_POINT('Ctrl Pts',(-68.3451482241569,0.000196976755690901,
38.4986596531413));
#23383=CARTESIAN_POINT('Ctrl Pts',(-68.3458954542973,0.000180736347680724,
38.4966133355963));
#23384=CARTESIAN_POINT('Ctrl Pts',(-68.3466257050307,0.000165866018364547,
38.4946135036599));
#23385=CARTESIAN_POINT('Ctrl Pts',(-68.3472620355198,0.000152908217028115,
38.4928708774956));
#23386=CARTESIAN_POINT('Ctrl Pts',(-68.3478852314339,0.000140979676548259,
38.4911642110139));
#23387=CARTESIAN_POINT('Ctrl Pts',(-68.3484914173096,0.000130049360615558,
38.4895041189565));
#23388=CARTESIAN_POINT('Ctrl Pts',(-68.3490583867176,0.000119826168353269,
38.4879514245622));
#23389=CARTESIAN_POINT('Ctrl Pts',(-68.3496102868861,0.000110468347365426,
38.4864399907313));
#23390=CARTESIAN_POINT('Ctrl Pts',(-68.35015981844,0.000101705602237878,
38.4849350380393));
#23391=CARTESIAN_POINT('Ctrl Pts',(-68.3507102521346,9.2928471713106E-5,
38.4834276147353));
#23392=CARTESIAN_POINT('Ctrl Pts',(-68.3512614066828,8.4698082740561E-5,
38.4819182119414));
#23393=CARTESIAN_POINT('Ctrl Pts',(-68.3518273692186,7.68530577763826E-5,
38.4803682529445));
#23394=CARTESIAN_POINT('Ctrl Pts',(-68.3524400983118,6.83597835248359E-5,
38.4786902178969));
#23395=CARTESIAN_POINT('Ctrl Pts',(-68.3530700017665,6.03342623984873E-5,
38.4769651454958));
#23396=CARTESIAN_POINT('Ctrl Pts',(-68.3537140995719,5.292526822398E-5,
38.475201198733));
#23397=CARTESIAN_POINT('Ctrl Pts',(-68.3544669502882,4.42652999317775E-5,
38.4731394177847));
#23398=CARTESIAN_POINT('Ctrl Pts',(-68.3552388964745,3.64757767242872E-5,
38.4710253395818));
#23399=CARTESIAN_POINT('Ctrl Pts',(-68.356001069178,2.98874821691442E-5,
38.4689380276888));
#23400=CARTESIAN_POINT('Ctrl Pts',(-68.3569159940322,2.19787832524977E-5,
38.4664323836002));
#23401=CARTESIAN_POINT('Ctrl Pts',(-68.3578152159407,1.58466561415058E-5,
38.4639697446387));
#23402=CARTESIAN_POINT('Ctrl Pts',(-68.3586312278135,1.14758455520558E-5,
38.4617349910484));
#23403=CARTESIAN_POINT('Ctrl Pts',(-68.3592601968496,8.10689392889741E-6,
38.4600124783516));
#23404=CARTESIAN_POINT('Ctrl Pts',(-68.3598389430335,5.75949590045699E-6,
38.4584275097792));
#23405=CARTESIAN_POINT('Ctrl Pts',(-68.3603434551658,4.13699435153347E-6,
38.4570458438162));
#23406=CARTESIAN_POINT('Ctrl Pts',(-68.3608017388602,2.66316259131356E-6,
38.4557907798814));
#23407=CARTESIAN_POINT('Ctrl Pts',(-68.3611984502224,1.7762057194213E-6,
38.454704342253));
#23408=CARTESIAN_POINT('Ctrl Pts',(-68.3615283751663,1.20384661084216E-6,
38.4538008101588));
#23409=CARTESIAN_POINT('Ctrl Pts',(-68.3618379571167,6.66778855064765E-7,
38.4529529893644));
#23410=CARTESIAN_POINT('Ctrl Pts',(-68.3620885334905,4.02530356487505E-7,
38.4522667649716));
#23411=CARTESIAN_POINT('Ctrl Pts',(-68.3622911397606,2.44220873746315E-7,
38.4517119142492));
#23412=CARTESIAN_POINT('Ctrl Pts',(-68.3624807302953,9.6081433271387E-8,
38.4511927079823));
#23413=CARTESIAN_POINT('Ctrl Pts',(-68.3626282304319,4.1248889315617E-8,
38.4507887728746));
#23414=CARTESIAN_POINT('Ctrl Pts',(-68.3627584528418,1.55631951770374E-8,
38.4504321554389));
#23415=CARTESIAN_POINT('Ctrl Pts',(-68.3628129524137,4.81343762933541E-9,
38.4502829069525));
#23416=CARTESIAN_POINT('Ctrl Pts',(-68.3628646310447,1.77646490962825E-15,
38.4501413840425));
#23417=CARTESIAN_POINT('Ctrl Pts',(-68.3629162589689,1.77635683940025E-15,
38.45));
#23418=CARTESIAN_POINT('',(-68.2564581294845,1.38777878078145E-15,38.1584524052577));
#23419=CARTESIAN_POINT('Ctrl Pts',(-68.337524038529,5.93046172356853,44.4495970221433));
#23420=CARTESIAN_POINT('Ctrl Pts',(-68.3380554670654,5.93191700291027,44.4496138895457));
#23421=CARTESIAN_POINT('Ctrl Pts',(-68.33972470056,5.93648800368254,44.4496722893984));
#23422=CARTESIAN_POINT('Ctrl Pts',(-68.3466592038245,5.95547810050877,44.449843145505));
#23423=CARTESIAN_POINT('Ctrl Pts',(-68.3522696681409,5.97084299769377,44.4499400860122));
#23424=CARTESIAN_POINT('Ctrl Pts',(-68.3583197127975,5.98741189639329,44.4499921112246));
#23425=CARTESIAN_POINT('Ctrl Pts',(-68.3618851430649,5.99717624795805,44.4500002303499));
#23426=CARTESIAN_POINT('Ctrl Pts',(-68.3625619515145,5.99902972236498,44.45));
#23427=CARTESIAN_POINT('Ctrl Pts',(-68.3629162589689,6.,44.45));
#23428=CARTESIAN_POINT('Ctrl Pts',(-68.2126657709715,5.97605464977923,44.4423397416413));
#23429=CARTESIAN_POINT('Ctrl Pts',(-68.2143126524885,5.98062783486323,44.4424272990272));
#23430=CARTESIAN_POINT('Ctrl Pts',(-68.2207643044116,5.99843724151488,44.4431085011719));
#23431=CARTESIAN_POINT('Ctrl Pts',(-68.2398084203356,6.05086488453047,44.445030680802));
#23432=CARTESIAN_POINT('Ctrl Pts',(-68.2597610177883,6.1057974519237,44.447239609276));
#23433=CARTESIAN_POINT('Ctrl Pts',(-68.277199866261,6.15377628468129,44.4488972071928));
#23434=CARTESIAN_POINT('Ctrl Pts',(-68.2878612524352,6.18311475992958,44.449788194713));
#23435=CARTESIAN_POINT('Ctrl Pts',(-68.2908360008298,6.19131037030115,44.45));
#23436=CARTESIAN_POINT('Ctrl Pts',(-68.291944172646,6.19436506316151,44.45));
#23437=CARTESIAN_POINT('Ctrl Pts',(-68.0878075034141,6.02164757598992,44.4350824611393));
#23438=CARTESIAN_POINT('Ctrl Pts',(-68.0905626050853,6.02935582072253,44.4354729132527));
#23439=CARTESIAN_POINT('Ctrl Pts',(-68.0980970765099,6.0500556176474,44.4375085746815));
#23440=CARTESIAN_POINT('Ctrl Pts',(-68.1376006723052,6.15744101353435,44.4426124063033));
#23441=CARTESIAN_POINT('Ctrl Pts',(-68.1645086369594,6.23181080403112,44.4468591341426));
#23442=CARTESIAN_POINT('Ctrl Pts',(-68.1976137828852,6.32327377665533,44.4489683068506));
#23443=CARTESIAN_POINT('Ctrl Pts',(-68.216530184342,6.3761496036587,44.4495903553226));
#23444=CARTESIAN_POINT('Ctrl Pts',(-68.219110050145,6.38359101823731,44.45));
#23445=CARTESIAN_POINT('Ctrl Pts',(-68.220972086323,6.38873012632302,44.45));
#23446=CARTESIAN_POINT('Ctrl Pts',(-67.9629492358566,6.06724050220062,44.4278251806373));
#23447=CARTESIAN_POINT('Ctrl Pts',(-67.9667888156612,6.07805539713409,44.4287485196527));
#23448=CARTESIAN_POINT('Ctrl Pts',(-67.9787581135963,6.11198288397358,44.4319313091104));
#23449=CARTESIAN_POINT('Ctrl Pts',(-68.0292786066066,6.25280322257157,44.4413031100688));
#23450=CARTESIAN_POINT('Ctrl Pts',(-68.0708345311172,6.36674803437274,44.4466862872856));
#23451=CARTESIAN_POINT('Ctrl Pts',(-68.1158705867169,6.48963058632797,44.449565613891));
#23452=CARTESIAN_POINT('Ctrl Pts',(-68.1423752254407,6.56208650902341,44.4500126088173));
#23453=CARTESIAN_POINT('Ctrl Pts',(-68.1473840994603,6.57587166617348,44.45));
#23454=CARTESIAN_POINT('Ctrl Pts',(-68.15,6.58309518948453,44.45));
#23455=CARTESIAN_POINT('',(-68.3629162589689,6.,44.45));
#23456=CARTESIAN_POINT('',(-68.337524038529,5.93046172356853,44.4495970221433));
#23457=CARTESIAN_POINT('Ctrl Pts',(-68.3629162589689,6.,44.45));
#23458=CARTESIAN_POINT('Ctrl Pts',(-68.3627923897953,5.99966078193582,44.45));
#23459=CARTESIAN_POINT('Ctrl Pts',(-68.3626669120248,5.99931715850946,44.449999977092));
#23460=CARTESIAN_POINT('Ctrl Pts',(-68.3625071684643,5.99887969292084,44.4499998954093));
#23461=CARTESIAN_POINT('Ctrl Pts',(-68.3623399907767,5.99842186860966,44.4499998099254));
#23462=CARTESIAN_POINT('Ctrl Pts',(-68.3621354236744,5.99786164759464,44.4499996610084));
#23463=CARTESIAN_POINT('Ctrl Pts',(-68.3618760240636,5.99715125894938,44.4499993237228));
#23464=CARTESIAN_POINT('Ctrl Pts',(-68.3615826009174,5.99634769386054,44.449998942198));
#23465=CARTESIAN_POINT('Ctrl Pts',(-68.3612190270722,5.99535200978922,44.4499983178149));
#23466=CARTESIAN_POINT('Ctrl Pts',(-68.3607842715223,5.99416138267066,44.4499971592116));
#23467=CARTESIAN_POINT('Ctrl Pts',(-68.3603085925964,5.99285868227063,44.4499958915495));
#23468=CARTESIAN_POINT('Ctrl Pts',(-68.359748146621,5.99132383303226,44.4499939695697));
#23469=CARTESIAN_POINT('Ctrl Pts',(-68.3591251743955,5.98961774472287,44.4499910173912));
#23470=CARTESIAN_POINT('Ctrl Pts',(-68.3581934848705,5.98706619500446,44.4499866022445));
#23471=CARTESIAN_POINT('Ctrl Pts',(-68.3571236235583,5.98413623755589,44.4499797759452));
#23472=CARTESIAN_POINT('Ctrl Pts',(-68.3560299762101,5.98114113800634,44.4499703618705));
#23473=CARTESIAN_POINT('Ctrl Pts',(-68.3552924432318,5.97912130529265,44.4499640132147));
#23474=CARTESIAN_POINT('Ctrl Pts',(-68.3545452035351,5.97707488911023,44.449956536428));
#23475=CARTESIAN_POINT('Ctrl Pts',(-68.3538149425036,5.97507497282754,44.4499482283617));
#23476=CARTESIAN_POINT('Ctrl Pts',(-68.3531786038672,5.97333227542841,44.4499409888359));
#23477=CARTESIAN_POINT('Ctrl Pts',(-68.3525553992048,5.97162554830819,44.4499331368466));
#23478=CARTESIAN_POINT('Ctrl Pts',(-68.3519492040121,5.96996540673227,44.449924826463));
#23479=CARTESIAN_POINT('Ctrl Pts',(-68.3513822292988,5.96841267535893,44.4499170537564));
#23480=CARTESIAN_POINT('Ctrl Pts',(-68.3508303231258,5.96690121361164,44.4499088939209));
#23481=CARTESIAN_POINT('Ctrl Pts',(-68.350280785426,5.96539624329614,44.4499002141721));
#23482=CARTESIAN_POINT('Ctrl Pts',(-68.3497303427571,5.96388879462198,44.4498915201296));
#23483=CARTESIAN_POINT('Ctrl Pts',(-68.3491791791713,5.96237937698876,44.4498822564462));
#23484=CARTESIAN_POINT('Ctrl Pts',(-68.3486132068006,5.9608294119577,44.4498721373903));
#23485=CARTESIAN_POINT('Ctrl Pts',(-68.3480004704559,5.95915137967762,44.4498611822383));
#23486=CARTESIAN_POINT('Ctrl Pts',(-68.3473705590191,5.95742632106119,44.4498492142267));
#23487=CARTESIAN_POINT('Ctrl Pts',(-68.3467264521375,5.95566239775521,44.4498361791825));
#23488=CARTESIAN_POINT('Ctrl Pts',(-68.3459735972113,5.95360066174812,44.4498209433613));
#23489=CARTESIAN_POINT('Ctrl Pts',(-68.3452016456489,5.95148664284324,44.449804231063));
#23490=CARTESIAN_POINT('Ctrl Pts',(-68.3444394655155,5.94939939730536,44.4497866277899));
#23491=CARTESIAN_POINT('Ctrl Pts',(-68.3435245038817,5.94689375657353,44.4497654958833));
#23492=CARTESIAN_POINT('Ctrl Pts',(-68.3426252430715,5.94443113354186,44.4497430857958));
#23493=CARTESIAN_POINT('Ctrl Pts',(-68.3418091957487,5.94219640517136,44.4497215555745));
#23494=CARTESIAN_POINT('Ctrl Pts',(-68.3411802068166,5.94047393225571,44.4497049606166));
#23495=CARTESIAN_POINT('Ctrl Pts',(-68.3406014416822,5.93888900549839,44.4496889382244));
#23496=CARTESIAN_POINT('Ctrl Pts',(-68.3400969132081,5.93750737818474,44.4496745471916));
#23497=CARTESIAN_POINT('Ctrl Pts',(-68.3396386155056,5.93625235164827,44.4496614748327));
#23498=CARTESIAN_POINT('Ctrl Pts',(-68.3392418920764,5.93516594802355,44.449649769955));
#23499=CARTESIAN_POINT('Ctrl Pts',(-68.338911958005,5.93426244474791,44.4496398703447));
#23500=CARTESIAN_POINT('Ctrl Pts',(-68.338602367729,5.93341465165008,44.4496305811462));
#23501=CARTESIAN_POINT('Ctrl Pts',(-68.338351785533,5.93272845006159,44.4496228920195));
#23502=CARTESIAN_POINT('Ctrl Pts',(-68.33814917651,5.93217361966125,44.4496166195958));
#23503=CARTESIAN_POINT('Ctrl Pts',(-68.3379595836667,5.93165443314326,44.4496107501304));
#23504=CARTESIAN_POINT('Ctrl Pts',(-68.3378120837905,5.93125051527315,44.4496061233657));
#23505=CARTESIAN_POINT('Ctrl Pts',(-68.3376818644882,5.93089391885477,44.4496020159298));
#23506=CARTESIAN_POINT('Ctrl Pts',(-68.3376273573399,5.93074465485525,44.4496002966407));
#23507=CARTESIAN_POINT('Ctrl Pts',(-68.3375756725639,5.93060311970978,44.449598660994));
#23508=CARTESIAN_POINT('Ctrl Pts',(-68.337524038529,5.93046172356853,44.4495970221433));
#23509=CARTESIAN_POINT('',(-67.9629492358566,6.06724050220062,44.4278251806373));
#23510=CARTESIAN_POINT('Ctrl Pts',(-67.9629492358566,6.06724050220062,44.4278251806373));
#23511=CARTESIAN_POINT('Ctrl Pts',(-68.0878075034141,6.02164757598992,44.4350824611393));
#23512=CARTESIAN_POINT('Ctrl Pts',(-68.2126657709715,5.97605464977923,44.4423397416413));
#23513=CARTESIAN_POINT('Ctrl Pts',(-68.337524038529,5.93046172356853,44.4495970221433));
#23514=CARTESIAN_POINT('',(-68.15,6.58309518948453,44.45));
#23515=CARTESIAN_POINT('Ctrl Pts',(-67.9629492358566,6.06724050220062,44.4278251806373));
#23516=CARTESIAN_POINT('Ctrl Pts',(-67.9634792046529,6.06873325847658,44.4279526271005));
#23517=CARTESIAN_POINT('Ctrl Pts',(-67.9640107571925,6.07023015560885,44.4280799229926));
#23518=CARTESIAN_POINT('Ctrl Pts',(-67.9645984647883,6.07188520707584,44.428219937255));
#23519=CARTESIAN_POINT('Ctrl Pts',(-67.9652135065932,6.07361723478624,44.4283664635638));
#23520=CARTESIAN_POINT('Ctrl Pts',(-67.9658900396361,6.07552244720398,44.4285269212262));
#23521=CARTESIAN_POINT('Ctrl Pts',(-67.9666715313615,6.07772300648473,44.4287109043712));
#23522=CARTESIAN_POINT('Ctrl Pts',(-67.9674818862731,6.0800048400133,44.4289016826487));
#23523=CARTESIAN_POINT('Ctrl Pts',(-67.9684050288702,6.08260405096595,44.4291177455802));
#23524=CARTESIAN_POINT('Ctrl Pts',(-67.9694699998137,6.08560145945498,44.4293644327481));
#23525=CARTESIAN_POINT('Ctrl Pts',(-67.9705830508425,6.08873419150098,44.4296222570649));
#23526=CARTESIAN_POINT('Ctrl Pts',(-67.9718509454418,6.0923016544676,44.4299135097813));
#23527=CARTESIAN_POINT('Ctrl Pts',(-67.9732871132029,6.09633987852639,44.4302387811688));
#23528=CARTESIAN_POINT('Ctrl Pts',(-67.9748066016361,6.10061238408877,44.4305829234929));
#23529=CARTESIAN_POINT('Ctrl Pts',(-67.9765143547191,6.10541155386422,44.4309650964591));
#23530=CARTESIAN_POINT('Ctrl Pts',(-67.9784060294667,6.11072251487592,44.4313805150352));
#23531=CARTESIAN_POINT('Ctrl Pts',(-67.9804509378605,6.11646368616668,44.4318295842709));
#23532=CARTESIAN_POINT('Ctrl Pts',(-67.9827106320591,6.1228024800746,44.4323174065272));
#23533=CARTESIAN_POINT('Ctrl Pts',(-67.9851583897365,6.12966028043662,44.4328328324271));
#23534=CARTESIAN_POINT('Ctrl Pts',(-67.9879348778881,6.1374390739121,44.4334174793131));
#23535=CARTESIAN_POINT('Ctrl Pts',(-67.9909530856534,6.1458848393196,44.4340374388882));
#23536=CARTESIAN_POINT('Ctrl Pts',(-67.9941504668408,6.15481772771674,44.4346724941108));
#23537=CARTESIAN_POINT('Ctrl Pts',(-67.9991033815213,6.16865525020394,44.4356562286581));
#23538=CARTESIAN_POINT('Ctrl Pts',(-68.0044847691739,6.18365673017047,44.4366745490167));
#23539=CARTESIAN_POINT('Ctrl Pts',(-68.0100131590845,6.19902659071492,44.4376570855204));
#23540=CARTESIAN_POINT('Ctrl Pts',(-68.0135448047944,6.20884516410302,44.4382847494306));
#23541=CARTESIAN_POINT('Ctrl Pts',(-68.0171353174438,6.21881124266636,44.4388980670586));
#23542=CARTESIAN_POINT('Ctrl Pts',(-68.0207185807072,6.22874060154588,44.4394848412893));
#23543=CARTESIAN_POINT('Ctrl Pts',(-68.0240778900166,6.23804937549544,44.4400349421306));
#23544=CARTESIAN_POINT('Ctrl Pts',(-68.0274303123981,6.24732450256424,44.4405617369221));
#23545=CARTESIAN_POINT('Ctrl Pts',(-68.0307378123003,6.25646133483194,44.4410603836529));
#23546=CARTESIAN_POINT('Ctrl Pts',(-68.0336280436266,6.26444547984301,44.4414961219582));
#23547=CARTESIAN_POINT('Ctrl Pts',(-68.0364839523164,6.27232401047471,44.4419104549468));
#23548=CARTESIAN_POINT('Ctrl Pts',(-68.0392959553735,6.28007146409556,44.442303360149));
#23549=CARTESIAN_POINT('Ctrl Pts',(-68.0419389442854,6.28735326059455,44.4426726499654));
#23550=CARTESIAN_POINT('Ctrl Pts',(-68.044543054373,6.29451902765292,44.4430230546008));
#23551=CARTESIAN_POINT('Ctrl Pts',(-68.0471162156862,6.30159180110784,44.4433567463161));
#23552=CARTESIAN_POINT('Ctrl Pts',(-68.0495855904277,6.30837929944029,44.4436769788212));
#23553=CARTESIAN_POINT('Ctrl Pts',(-68.0520263717406,6.31508091627373,44.4439818551754));
#23554=CARTESIAN_POINT('Ctrl Pts',(-68.0544620138325,6.32176249132158,44.4442748222115));
#23555=CARTESIAN_POINT('Ctrl Pts',(-68.0569473578197,6.32858041109119,44.4445737675549));
#23556=CARTESIAN_POINT('Ctrl Pts',(-68.0594301387449,6.33538518337142,44.4448606695783));
#23557=CARTESIAN_POINT('Ctrl Pts',(-68.0619414059941,6.34226352245981,44.4451387828686));
#23558=CARTESIAN_POINT('Ctrl Pts',(-68.064532863982,6.34936150328192,44.445425776978));
#23559=CARTESIAN_POINT('Ctrl Pts',(-68.0671545943889,6.35653763294209,44.445703347439));
#23560=CARTESIAN_POINT('Ctrl Pts',(-68.0698203494605,6.36383078703253,44.4459718736484));
#23561=CARTESIAN_POINT('Ctrl Pts',(-68.0726342429007,6.37152922815088,44.446255322097));
#23562=CARTESIAN_POINT('Ctrl Pts',(-68.0754970824222,6.37935774693701,44.4465286150822));
#23563=CARTESIAN_POINT('Ctrl Pts',(-68.0784041665278,6.38730452967628,44.4467898321574));
#23564=CARTESIAN_POINT('Ctrl Pts',(-68.0815330051503,6.39585749885638,44.4470709750635));
#23565=CARTESIAN_POINT('Ctrl Pts',(-68.0847129375142,6.40454701081627,44.4473380241526));
#23566=CARTESIAN_POINT('Ctrl Pts',(-68.0879165455132,6.41329920716382,44.447587389995));
#23567=CARTESIAN_POINT('Ctrl Pts',(-68.0915250570896,6.4231575924126,44.4478682731521));
#23568=CARTESIAN_POINT('Ctrl Pts',(-68.0951633311916,6.43309474069371,44.4481265525169));
#23569=CARTESIAN_POINT('Ctrl Pts',(-68.0987689579151,6.44294165688685,44.4483579274529));
#23570=CARTESIAN_POINT('Ctrl Pts',(-68.1055598239949,6.46148741724862,44.4487937008497));
#23571=CARTESIAN_POINT('Ctrl Pts',(-68.1122324839575,6.47970668562001,44.4491309639825));
#23572=CARTESIAN_POINT('Ctrl Pts',(-68.118284360492,6.49623650829922,44.4493710766663));
#23573=CARTESIAN_POINT('Ctrl Pts',(-68.1213794941395,6.50469041678024,44.4494938783861));
#23574=CARTESIAN_POINT('Ctrl Pts',(-68.1243116528742,6.51270076758936,44.4495920666801));
#23575=CARTESIAN_POINT('Ctrl Pts',(-68.1270242533871,6.52011386974791,44.4496700038563));
#23576=CARTESIAN_POINT('Ctrl Pts',(-68.1294687572352,6.52679430671845,44.4497402382039));
#23577=CARTESIAN_POINT('Ctrl Pts',(-68.1317347258717,6.53298908188991,44.4497941150971));
#23578=CARTESIAN_POINT('Ctrl Pts',(-68.133795075469,6.538624477974,44.4498358584241));
#23579=CARTESIAN_POINT('Ctrl Pts',(-68.1357220174723,6.54389498227775,44.4498748988714));
#23580=CARTESIAN_POINT('Ctrl Pts',(-68.1374689566185,6.54867578880567,44.4499033746776));
#23581=CARTESIAN_POINT('Ctrl Pts',(-68.1390295368681,6.55294946200119,44.4499247770501));
#23582=CARTESIAN_POINT('Ctrl Pts',(-68.1404811145484,6.55692462997174,44.4499446845213));
#23583=CARTESIAN_POINT('Ctrl Pts',(-68.1417714173016,6.56046091928347,44.4499584916947));
#23584=CARTESIAN_POINT('Ctrl Pts',(-68.1429106739614,6.56358602529867,44.4499685877935));
#23585=CARTESIAN_POINT('Ctrl Pts',(-68.1440153840732,6.56661636634192,44.4499783777406));
#23586=CARTESIAN_POINT('Ctrl Pts',(-68.144977967085,6.56925979952851,44.4499846840721));
#23587=CARTESIAN_POINT('Ctrl Pts',(-68.1458238660412,6.57158547767846,44.4499890998665));
#23588=CARTESIAN_POINT('Ctrl Pts',(-68.1466475415774,6.57385005571468,44.4499933996493));
#23589=CARTESIAN_POINT('Ctrl Pts',(-68.1473604970041,6.57581311688528,44.4499959037341));
#23590=CARTESIAN_POINT('Ctrl Pts',(-68.1480031204066,6.57758458469693,44.4499975077911));
#23591=CARTESIAN_POINT('Ctrl Pts',(-68.1486256515068,6.57930066568863,44.4499990616955));
#23592=CARTESIAN_POINT('Ctrl Pts',(-68.1491821314357,6.58083681318181,44.4499997670013));
#23593=CARTESIAN_POINT('Ctrl Pts',(-68.149726292367,6.58233938708418,44.4499999531776));
#23594=CARTESIAN_POINT('Ctrl Pts',(-68.1498177332245,6.58259187975336,44.4499999844627));
#23595=CARTESIAN_POINT('Ctrl Pts',(-68.1499088672424,6.58284353633912,44.45));
#23596=CARTESIAN_POINT('Ctrl Pts',(-68.15,6.58309518948453,44.45));
#23597=CARTESIAN_POINT('',(-68.2564581294845,6.29154759474226,44.45));
#23598=CARTESIAN_POINT('Ctrl Pts',(-67.9629492358566,6.06724050220062,44.4278251806372));
#23599=CARTESIAN_POINT('Ctrl Pts',(-67.6593813620821,5.21218478592245,44.3548234262939));
#23600=CARTESIAN_POINT('Ctrl Pts',(-67.3499999997967,4.23816712577606,44.060861613326));
#23601=CARTESIAN_POINT('Ctrl Pts',(-67.35,3.42868316199151,43.6499999996042));
#23602=CARTESIAN_POINT('Ctrl Pts',(-68.0878075034141,6.02164757598992,44.4350824611393));
#23603=CARTESIAN_POINT('Ctrl Pts',(-67.7813554130122,5.16661251454587,44.3831113590611));
#23604=CARTESIAN_POINT('Ctrl Pts',(-67.4526591694531,4.19555805202367,44.1114585399875));
#23605=CARTESIAN_POINT('Ctrl Pts',(-67.4229730822988,3.3926665294012,43.7061729265265));
#23606=CARTESIAN_POINT('Ctrl Pts',(-68.2126657709715,5.97605464977923,44.4423397416413));
#23607=CARTESIAN_POINT('Ctrl Pts',(-67.9033294639424,5.12104024316929,44.4113992918283));
#23608=CARTESIAN_POINT('Ctrl Pts',(-67.5553183391094,4.15294897827129,44.162055466649));
#23609=CARTESIAN_POINT('Ctrl Pts',(-67.4959461645976,3.35664989681088,43.7623458534489));
#23610=CARTESIAN_POINT('Ctrl Pts',(-68.337524038529,5.93046172356853,44.4495970221433));
#23611=CARTESIAN_POINT('Ctrl Pts',(-68.0253035148726,5.07546797179271,44.4396872245955));
#23612=CARTESIAN_POINT('Ctrl Pts',(-67.6579775087658,4.1103399045189,44.2126523933104));
#23613=CARTESIAN_POINT('Ctrl Pts',(-67.5689192468964,3.32063326422057,43.8185187803712));
#23614=CARTESIAN_POINT('',(-67.5689192468964,3.32063326422069,43.8185187803713));
#23615=CARTESIAN_POINT('Ctrl Pts',(-68.337524038529,5.93046172356853,44.4495970221433));
#23616=CARTESIAN_POINT('Ctrl Pts',(-68.0253035148726,5.07546797179271,44.4396872245955));
#23617=CARTESIAN_POINT('Ctrl Pts',(-67.6579775087658,4.1103399045189,44.2126523933104));
#23618=CARTESIAN_POINT('Ctrl Pts',(-67.5689192468964,3.32063326422057,43.8185187803712));
#23619=CARTESIAN_POINT('',(-67.35,3.42868316190267,43.6499999997796));
#23620=CARTESIAN_POINT('',(-67.5689192468964,3.32063326422069,43.8185187803713));
#23621=CARTESIAN_POINT('Ctrl Pts',(-67.35,3.42868316199151,43.6499999996042));
#23622=CARTESIAN_POINT('Ctrl Pts',(-67.3499999997967,4.23816712577606,44.060861613326));
#23623=CARTESIAN_POINT('Ctrl Pts',(-67.6593813620821,5.21218478592245,44.3548234262939));
#23624=CARTESIAN_POINT('Ctrl Pts',(-67.9629492358566,6.06724050220062,44.4278251806372));
#23625=CARTESIAN_POINT('Origin',(-67.45,6.00000000000001,38.45));
#23626=CARTESIAN_POINT('',(-67.55,0.800000000000003,41.4433259094192));
#23627=CARTESIAN_POINT('',(-67.35,0.973333333333333,41.3435483791052));
#23628=CARTESIAN_POINT('',(-67.55,0.800000000000003,41.4433259094192));
#23629=CARTESIAN_POINT('',(-67.35,3.10645162089482,43.4766666666667));
#23630=CARTESIAN_POINT('Origin',(-67.35,6.00000000000001,38.45));
#23631=CARTESIAN_POINT('',(-67.55,3.00667409058085,43.65));
#23632=CARTESIAN_POINT('',(-67.35,3.10645162089482,43.4766666666667));
#23633=CARTESIAN_POINT('Origin',(-67.55,6.00000000000001,38.45));
#23634=CARTESIAN_POINT('Ctrl Pts',(-67.35,3.42868316199163,43.6499999996043));
#23635=CARTESIAN_POINT('Ctrl Pts',(-67.35,3.31801931336448,43.593831465749));
#23636=CARTESIAN_POINT('Ctrl Pts',(-67.35,3.2106959818173,43.5366738486782));
#23637=CARTESIAN_POINT('Ctrl Pts',(-67.35,3.10645162089482,43.4766666666667));
#23638=CARTESIAN_POINT('Ctrl Pts',(-67.4229730822988,3.39266652940132,43.7061729265266));
#23639=CARTESIAN_POINT('Ctrl Pts',(-67.4189147231253,3.28290392767114,43.650766682816));
#23640=CARTESIAN_POINT('Ctrl Pts',(-67.4166666666667,3.17639835547357,43.5938538537616));
#23641=CARTESIAN_POINT('Ctrl Pts',(-67.4166666666667,3.0731924441235,43.5344444444444));
#23642=CARTESIAN_POINT('Ctrl Pts',(-67.4959461645976,3.356649896811,43.7623458534489));
#23643=CARTESIAN_POINT('Ctrl Pts',(-67.4878294462506,3.24778854197779,43.7077018998829));
#23644=CARTESIAN_POINT('Ctrl Pts',(-67.4833333333333,3.14210072912983,43.651033858845));
#23645=CARTESIAN_POINT('Ctrl Pts',(-67.4833333333333,3.03993326735218,43.5922222222222));
#23646=CARTESIAN_POINT('Ctrl Pts',(-67.5689192468964,3.32063326422068,43.8185187803713));
#23647=CARTESIAN_POINT('Ctrl Pts',(-67.556744169376,3.21267315628445,43.7646371169499));
#23648=CARTESIAN_POINT('Ctrl Pts',(-67.55,3.1078031027861,43.7082138639284));
#23649=CARTESIAN_POINT('Ctrl Pts',(-67.55,3.00667409058085,43.65));
#23650=CARTESIAN_POINT('Ctrl Pts',(-67.35,3.10645162089482,43.4766666666667));
#23651=CARTESIAN_POINT('Ctrl Pts',(-67.35,3.2106959818173,43.5366738486782));
#23652=CARTESIAN_POINT('Ctrl Pts',(-67.35,3.31801931336448,43.593831465749));
#23653=CARTESIAN_POINT('Ctrl Pts',(-67.35,3.42868316199163,43.6499999996043));
#23654=CARTESIAN_POINT('Ctrl Pts',(-67.5689192468964,3.32063326422068,43.8185187803713));
#23655=CARTESIAN_POINT('Ctrl Pts',(-67.556744169376,3.21267315628445,43.7646371169499));
#23656=CARTESIAN_POINT('Ctrl Pts',(-67.55,3.1078031027861,43.7082138639284));
#23657=CARTESIAN_POINT('Ctrl Pts',(-67.55,3.00667409058085,43.65));
#23658=CARTESIAN_POINT('Ctrl Pts',(-67.35,0.800000000395797,41.0213168380085));
#23659=CARTESIAN_POINT('Ctrl Pts',(-67.3499999997967,0.389138161249131,
40.2118324300895));
#23660=CARTESIAN_POINT('Ctrl Pts',(-67.6593820111175,0.0951762114108467,
39.2378132607964));
#23661=CARTESIAN_POINT('Ctrl Pts',(-67.9629497353532,0.0221746992443747,
38.3827580908662));
#23662=CARTESIAN_POINT('Ctrl Pts',(-67.4229730822988,0.743827073473452,
41.0573334705988));
#23663=CARTESIAN_POINT('Ctrl Pts',(-67.4526591857407,0.33854123764703,40.254441507459));
#23664=CARTESIAN_POINT('Ctrl Pts',(-67.7813558695995,0.0668883318015427,
39.2833861208106));
#23665=CARTESIAN_POINT('Ctrl Pts',(-68.0878080077738,0.014917453342854,
38.4283510167895));
#23666=CARTESIAN_POINT('Ctrl Pts',(-67.4959461645976,0.687654146551107,
41.0933501031891));
#23667=CARTESIAN_POINT('Ctrl Pts',(-67.5553183716848,0.287944314044929,
40.2970505848284));
#23668=CARTESIAN_POINT('Ctrl Pts',(-67.9033297280813,0.038600452192239,
39.3289589808248));
#23669=CARTESIAN_POINT('Ctrl Pts',(-68.2126662801944,0.00766020744133335,
38.4739439427128));
#23670=CARTESIAN_POINT('Ctrl Pts',(-67.5689192468964,0.631481219628762,
41.1293667357794));
#23671=CARTESIAN_POINT('Ctrl Pts',(-67.6579775576288,0.237347390442828,
40.3396596621978));
#23672=CARTESIAN_POINT('Ctrl Pts',(-68.0253035865633,0.0103125725829351,
39.374531840839));
#23673=CARTESIAN_POINT('Ctrl Pts',(-68.337524552615,0.000402961539812674,
38.5195368686361));
#23674=CARTESIAN_POINT('',(-67.35,0.800000000220445,41.0213168380973));
#23675=CARTESIAN_POINT('Ctrl Pts',(-67.9629497353532,0.0221746992443747,
38.3827580908662));
#23676=CARTESIAN_POINT('Ctrl Pts',(-67.6593820111175,0.0951762114108467,
39.2378132607964));
#23677=CARTESIAN_POINT('Ctrl Pts',(-67.3499999997967,0.389138161249131,
40.2118324300895));
#23678=CARTESIAN_POINT('Ctrl Pts',(-67.35,0.800000000395797,41.0213168380085));
#23679=CARTESIAN_POINT('',(-67.5689192468964,0.631481219628701,41.1293667357793));
#23680=CARTESIAN_POINT('',(-67.35,0.800000000220445,41.0213168380973));
#23681=CARTESIAN_POINT('Ctrl Pts',(-67.5689192468964,0.631481219628762,
41.1293667357794));
#23682=CARTESIAN_POINT('Ctrl Pts',(-67.6579775576288,0.237347390442828,
40.3396596621978));
#23683=CARTESIAN_POINT('Ctrl Pts',(-68.0253035865633,0.0103125725829351,
39.374531840839));
#23684=CARTESIAN_POINT('Ctrl Pts',(-68.337524552615,0.000402961539812674,
38.5195368686361));
#23685=CARTESIAN_POINT('Ctrl Pts',(-67.35,0.973333333333337,41.3435483791052));
#23686=CARTESIAN_POINT('Ctrl Pts',(-67.35,0.913326151321777,41.2393040181827));
#23687=CARTESIAN_POINT('Ctrl Pts',(-67.35,0.856168534250961,41.1319806866355));
#23688=CARTESIAN_POINT('Ctrl Pts',(-67.35,0.800000000395731,41.0213168380083));
#23689=CARTESIAN_POINT('Ctrl Pts',(-67.4166666666667,0.915555555555558,
41.3768075558765));
#23690=CARTESIAN_POINT('Ctrl Pts',(-67.4166666666667,0.856146146238368,
41.2736016445264));
#23691=CARTESIAN_POINT('Ctrl Pts',(-67.4189147231253,0.799233317184012,
41.1670960723288));
#23692=CARTESIAN_POINT('Ctrl Pts',(-67.4229730822988,0.743827073473387,
41.0573334705987));
#23693=CARTESIAN_POINT('Ctrl Pts',(-67.4833333333333,0.85777777777778,41.4100667326478));
#23694=CARTESIAN_POINT('Ctrl Pts',(-67.4833333333333,0.798966141154958,
41.3078992708702));
#23695=CARTESIAN_POINT('Ctrl Pts',(-67.4878294462506,0.742298100117064,
41.2022114580222));
#23696=CARTESIAN_POINT('Ctrl Pts',(-67.4959461645976,0.687654146551043,
41.093350103189));
#23697=CARTESIAN_POINT('Ctrl Pts',(-67.55,0.800000000000002,41.4433259094191));
#23698=CARTESIAN_POINT('Ctrl Pts',(-67.55,0.741786136071548,41.3421968972139));
#23699=CARTESIAN_POINT('Ctrl Pts',(-67.556744169376,0.685362883050115,41.2373268437155));
#23700=CARTESIAN_POINT('Ctrl Pts',(-67.5689192468964,0.6314812196287,41.1293667357793));
#23701=CARTESIAN_POINT('Ctrl Pts',(-67.35,0.800000000395731,41.0213168380083));
#23702=CARTESIAN_POINT('Ctrl Pts',(-67.35,0.856168534250961,41.1319806866355));
#23703=CARTESIAN_POINT('Ctrl Pts',(-67.35,0.913326151321777,41.2393040181827));
#23704=CARTESIAN_POINT('Ctrl Pts',(-67.35,0.973333333333337,41.3435483791052));
#23705=CARTESIAN_POINT('Ctrl Pts',(-67.55,0.800000000000002,41.4433259094191));
#23706=CARTESIAN_POINT('Ctrl Pts',(-67.55,0.741786136071548,41.3421968972139));
#23707=CARTESIAN_POINT('Ctrl Pts',(-67.556744169376,0.685362883050115,41.2373268437155));
#23708=CARTESIAN_POINT('Ctrl Pts',(-67.5689192468964,0.6314812196287,41.1293667357793));
#23709=CARTESIAN_POINT('Origin',(-67.35,6.,44.45));
#23710=CARTESIAN_POINT('',(-68.15,121.,44.45));
#23711=CARTESIAN_POINT('',(-68.15,34.75,44.45));
#23712=CARTESIAN_POINT('',(-71.3125,121.,44.45));
#23713=CARTESIAN_POINT('',(-67.35,121.,44.45));
#23714=CARTESIAN_POINT('',(-71.3125,6.58309518948451,44.45));
#23715=CARTESIAN_POINT('',(-71.3125,34.75,44.45));
#23716=CARTESIAN_POINT('',(-71.099583741031,6.,44.45));
#23717=CARTESIAN_POINT('',(-71.2060418705155,6.29154759474225,44.45));
#23718=CARTESIAN_POINT('',(-67.35,6.,44.45));
#23719=CARTESIAN_POINT('Origin',(-68.15,34.75,43.65));
#23720=CARTESIAN_POINT('',(-67.35,123.993325909419,43.65));
#23721=CARTESIAN_POINT('',(-67.35,34.75,43.65));
#23722=CARTESIAN_POINT('Ctrl Pts',(-67.35,123.993325909419,43.65));
#23723=CARTESIAN_POINT('Ctrl Pts',(-67.35,123.544851663295,43.9081595347366));
#23724=CARTESIAN_POINT('Ctrl Pts',(-67.4681119224052,123.043713064318,44.1162803662604));
#23725=CARTESIAN_POINT('Ctrl Pts',(-67.7780133341431,122.014025751789,44.387608349819));
#23726=CARTESIAN_POINT('Ctrl Pts',(-67.9725091568851,121.486078692623,44.45));
#23727=CARTESIAN_POINT('Ctrl Pts',(-68.15,121.,44.45));
#23728=CARTESIAN_POINT('Origin',(-67.35,63.5,-31.75));
#23729=CARTESIAN_POINT('',(-67.35,126.2,-104.943325909419));
#23730=CARTESIAN_POINT('Origin',(-67.35,121.,-101.95));
#23731=CARTESIAN_POINT('',(-67.35,126.2,41.4433259094192));
#23732=CARTESIAN_POINT('',(-67.35,126.2,3.35000000000001));
#23733=CARTESIAN_POINT('Origin',(-67.35,121.,38.45));
#23734=CARTESIAN_POINT('',(-67.35,0.800000000000001,-66.85));
#23735=CARTESIAN_POINT('Ctrl Pts',(-71.4995502644831,0.0221746992050148,
-101.882758090412));
#23736=CARTESIAN_POINT('Ctrl Pts',(-71.4893114115449,0.0197124751707447,
-101.853918449787));
#23737=CARTESIAN_POINT('Ctrl Pts',(-71.3975368407587,-0.000373182785439377,
-101.597454849766));
#23738=CARTESIAN_POINT('Ctrl Pts',(-71.320347680068,4.16333634234434E-16,
-101.388575320937));
#23739=CARTESIAN_POINT('Ctrl Pts',(-71.3125,4.16333634234434E-16,-101.366904810515));
#23740=CARTESIAN_POINT('Ctrl Pts',(-71.3746919921718,0.0149174533183786,
-101.928351016639));
#23741=CARTESIAN_POINT('Ctrl Pts',(-71.367345081829,0.0138762572832023,
-101.907795776398));
#23742=CARTESIAN_POINT('Ctrl Pts',(-71.3026241804508,-0.00241774122426398,
-101.725936069398));
#23743=CARTESIAN_POINT('Ctrl Pts',(-71.2471140006721,2.77555756156289E-16,
-101.576687138621));
#23744=CARTESIAN_POINT('Ctrl Pts',(-71.241527913677,2.77555756156289E-16,
-101.561269873677));
#23745=CARTESIAN_POINT('Ctrl Pts',(-71.2498337198606,0.00766020743174241,
-101.973943942866));
#23746=CARTESIAN_POINT('Ctrl Pts',(-71.2454420639835,0.00742672674743362,
-101.961748861474));
#23747=CARTESIAN_POINT('Ctrl Pts',(-71.2057787319611,0.00233147861827002,
-101.852535530178));
#23748=CARTESIAN_POINT('Ctrl Pts',(-71.1738803212761,1.38777878078145E-16,
-101.764798956304));
#23749=CARTESIAN_POINT('Ctrl Pts',(-71.170555827354,1.38777878078145E-16,
-101.755634936838));
#23750=CARTESIAN_POINT('Ctrl Pts',(-71.1249754475493,0.000402961545106217,
-102.019536869093));
#23751=CARTESIAN_POINT('Ctrl Pts',(-71.1235583334697,0.000357983626113174,
-102.01565620272));
#23752=CARTESIAN_POINT('Ctrl Pts',(-71.1109280101655,-7.85197747617509E-6,
-101.98106831054));
#23753=CARTESIAN_POINT('Ctrl Pts',(-71.1006466418801,-3.08148791101958E-32,
-101.952910773988));
#23754=CARTESIAN_POINT('Ctrl Pts',(-71.099583741031,-3.08148791101958E-32,
-101.95));
#23755=CARTESIAN_POINT('',(-71.3125,4.16333634234434E-16,-101.366904810515));
#23756=CARTESIAN_POINT('',(-71.4995502644831,0.0221746992050148,-101.882758090412));
#23757=CARTESIAN_POINT('Ctrl Pts',(-71.3125,5.55111512312578E-16,-101.366904810515));
#23758=CARTESIAN_POINT('Ctrl Pts',(-71.3130414730304,5.55111512312578E-16,
-101.368400029083));
#23759=CARTESIAN_POINT('Ctrl Pts',(-71.3135844616951,5.09286916164813E-7,
-101.369899384535));
#23760=CARTESIAN_POINT('Ctrl Pts',(-71.3141854581669,1.77548274082895E-6,
-101.371556771012));
#23761=CARTESIAN_POINT('Ctrl Pts',(-71.3148143991108,3.10055274469816E-6,
-101.373291220819));
#23762=CARTESIAN_POINT('Ctrl Pts',(-71.3155068597142,5.2499358755341E-6,
-101.375198716011));
#23763=CARTESIAN_POINT('Ctrl Pts',(-71.3163076848976,9.0615914953851E-6,
-101.377401328992));
#23764=CARTESIAN_POINT('Ctrl Pts',(-71.3171380744532,1.30139634765649E-5,
-101.379685256687));
#23765=CARTESIAN_POINT('Ctrl Pts',(-71.3180849092836,1.87480331671879E-5,
-101.382286305868));
#23766=CARTESIAN_POINT('Ctrl Pts',(-71.3191778991655,2.78719463189248E-5,
-101.385285246244));
#23767=CARTESIAN_POINT('Ctrl Pts',(-71.3203202081113,3.74075584838786E-5,
-101.388419508031));
#23768=CARTESIAN_POINT('Ctrl Pts',(-71.3216220759832,5.06497812803995E-5,
-101.391988146601));
#23769=CARTESIAN_POINT('Ctrl Pts',(-71.3230967976336,7.01856538209977E-5,
-101.396027187124));
#23770=CARTESIAN_POINT('Ctrl Pts',(-71.3246570195571,9.08541620961374E-5,
-101.400300400019));
#23771=CARTESIAN_POINT('Ctrl Pts',(-71.3264106102773,0.000118592480379773,
-101.405099836927));
#23772=CARTESIAN_POINT('Ctrl Pts',(-71.3283521800371,0.000157072677346992,
-101.410410677708));
#23773=CARTESIAN_POINT('Ctrl Pts',(-71.3304508784775,0.000198667025918302,
-101.416151317832));
#23774=CARTESIAN_POINT('Ctrl Pts',(-71.3327690542346,0.000252874495557993,
-101.422489045056));
#23775=CARTESIAN_POINT('Ctrl Pts',(-71.3352778797553,0.000324335624839467,
-101.429345386476));
#23776=CARTESIAN_POINT('Ctrl Pts',(-71.3381228078755,0.000405370266158498,
-101.437120258959));
#23777=CARTESIAN_POINT('Ctrl Pts',(-71.3412125993701,0.000508732077344889,
-101.445561210948));
#23778=CARTESIAN_POINT('Ctrl Pts',(-71.3444811993641,0.000639503798671726,
-101.454488825469));
#23779=CARTESIAN_POINT('Ctrl Pts',(-71.3495556162887,0.000842523512674709,
-101.468348716034));
#23780=CARTESIAN_POINT('Ctrl Pts',(-71.3550591995291,0.00111288776034773,
-101.483376639822));
#23781=CARTESIAN_POINT('Ctrl Pts',(-71.3606972637692,0.00145317997930938,
-101.498773355879));
#23782=CARTESIAN_POINT('Ctrl Pts',(-71.3642934091842,0.00167022970610506,
-101.508593894897));
#23783=CARTESIAN_POINT('Ctrl Pts',(-71.3679432157324,0.00191520565810608,
-101.518561639076));
#23784=CARTESIAN_POINT('Ctrl Pts',(-71.3715786877994,0.00218441438644557,
-101.528492379687));
#23785=CARTESIAN_POINT('Ctrl Pts',(-71.3749869428623,0.00243679756926383,
-101.53780244901));
#23786=CARTESIAN_POINT('Ctrl Pts',(-71.3783820993703,0.0027103343005662,
-101.547078622267));
#23787=CARTESIAN_POINT('Ctrl Pts',(-71.3817254092859,0.00300072602968982,
-101.556216272426));
#23788=CARTESIAN_POINT('Ctrl Pts',(-71.3846464362529,0.00325443929384036,
-101.564199774765));
#23789=CARTESIAN_POINT('Ctrl Pts',(-71.387527887852,0.00352092669085103,
-101.57207752597));
#23790=CARTESIAN_POINT('Ctrl Pts',(-71.3903601073981,0.00379788767176015,
-101.579824088709));
#23791=CARTESIAN_POINT('Ctrl Pts',(-71.3930216566499,0.00405815891116113,
-101.58710384154));
#23792=CARTESIAN_POINT('Ctrl Pts',(-71.3956396488113,0.00432761433456298,
-101.59426750665));
#23793=CARTESIAN_POINT('Ctrl Pts',(-71.3982220999012,0.00460593314475144,
-101.601338094212));
#23794=CARTESIAN_POINT('Ctrl Pts',(-71.400700919755,0.00487308329334014,
-101.608124946011));
#23795=CARTESIAN_POINT('Ctrl Pts',(-71.4031469125279,0.00514834328083419,
-101.614825801015));
#23796=CARTESIAN_POINT('Ctrl Pts',(-71.4055836015545,0.0054338019260769,
-101.621506457884));
#23797=CARTESIAN_POINT('Ctrl Pts',(-71.4080709217582,0.00572519202464918,
-101.628325929971));
#23798=CARTESIAN_POINT('Ctrl Pts',(-71.4105513407104,0.0060275143380851,
-101.635132076336));
#23799=CARTESIAN_POINT('Ctrl Pts',(-71.4130558783199,0.00634483852537349,
-101.642011678082));
#23800=CARTESIAN_POINT('Ctrl Pts',(-71.4156402620342,0.00667227919094947,
-101.649110605503));
#23801=CARTESIAN_POINT('Ctrl Pts',(-71.4182502522345,0.0070157417088504,
-101.656287555306));
#23802=CARTESIAN_POINT('Ctrl Pts',(-71.4208994927556,0.00737805356504495,
-101.663581424281));
#23803=CARTESIAN_POINT('Ctrl Pts',(-71.4236959576915,0.00776049992794052,
-101.671280630403));
#23804=CARTESIAN_POINT('Ctrl Pts',(-71.4265360348754,0.00816399914981401,
-101.679109796886));
#23805=CARTESIAN_POINT('Ctrl Pts',(-71.4294150279354,0.00858931252928419,
-101.687057097427));
#23806=CARTESIAN_POINT('Ctrl Pts',(-71.4325136453033,0.00904707098752052,
-101.695610658679));
#23807=CARTESIAN_POINT('Ctrl Pts',(-71.4356571655244,0.0095301632752057,
-101.704300612786));
#23808=CARTESIAN_POINT('Ctrl Pts',(-71.4388185948592,0.0100356890385436,
-101.713053049757));
#23809=CARTESIAN_POINT('Ctrl Pts',(-71.4423797356898,0.0106051303406133,
-101.722912090516));
#23810=CARTESIAN_POINT('Ctrl Pts',(-71.4459632961801,0.0112031338835822,
-101.73284964385));
#23811=CARTESIAN_POINT('Ctrl Pts',(-71.4495083874965,0.0118193723798979,
-101.742696590454));
#23812=CARTESIAN_POINT('Ctrl Pts',(-71.4561832840946,0.0129796607548892,
-101.761236973346));
#23813=CARTESIAN_POINT('Ctrl Pts',(-71.4627188234037,0.0142069874078384,
-101.779449700138));
#23814=CARTESIAN_POINT('Ctrl Pts',(-71.4686322703542,0.015383715339768,
-101.795972224294));
#23815=CARTESIAN_POINT('Ctrl Pts',(-71.4716575838855,0.0159857281699938,
-101.804425131087));
#23816=CARTESIAN_POINT('Ctrl Pts',(-71.474519665947,0.0165735928077044,
-101.812433997953));
#23817=CARTESIAN_POINT('Ctrl Pts',(-71.4771650469162,0.0171300093092834,
-101.819845063882));
#23818=CARTESIAN_POINT('Ctrl Pts',(-71.4795488917966,0.017631415588415,
-101.82652343338));
#23819=CARTESIAN_POINT('Ctrl Pts',(-71.481756561571,0.0181071458337637,
-101.832715726019));
#23820=CARTESIAN_POINT('Ctrl Pts',(-71.4837629698439,0.0185468695051121,
-101.838348235322));
#23821=CARTESIAN_POINT('Ctrl Pts',(-71.4856394395559,0.0189581158910569,
-101.843615973325));
#23822=CARTESIAN_POINT('Ctrl Pts',(-71.4873397382806,0.0193377870921649,
-101.848393672052));
#23823=CARTESIAN_POINT('Ctrl Pts',(-71.4888585891159,0.0196810600497634,
-101.852663957293));
#23824=CARTESIAN_POINT('Ctrl Pts',(-71.4902713548522,0.0200003568901358,
-101.856635981755));
#23825=CARTESIAN_POINT('Ctrl Pts',(-71.4915270995564,0.0202881342314904,
-101.86016888338));
#23826=CARTESIAN_POINT('Ctrl Pts',(-71.4926362824102,0.020544472237551,
-101.863290454269));
#23827=CARTESIAN_POINT('Ctrl Pts',(-71.493711825374,0.0207930358876558,
-101.86631735249));
#23828=CARTESIAN_POINT('Ctrl Pts',(-71.4946494637497,0.0210120087537537,
-101.868957207802));
#23829=CARTESIAN_POINT('Ctrl Pts',(-71.4954741507279,0.0212057651950597,
-101.871279309127));
#23830=CARTESIAN_POINT('Ctrl Pts',(-71.4962771686109,0.0213944305813664,
-101.873540395987));
#23831=CARTESIAN_POINT('Ctrl Pts',(-71.4969730084395,0.0215591700824165,
-101.875499969006));
#23832=CARTESIAN_POINT('Ctrl Pts',(-71.4976008832952,0.0217084974103041,
-101.877268125906));
#23833=CARTESIAN_POINT('Ctrl Pts',(-71.4982091346288,0.0218531576805589,
-101.878981021051));
#23834=CARTESIAN_POINT('Ctrl Pts',(-71.498753555179,0.0219833464849813,
-101.880514144293));
#23835=CARTESIAN_POINT('Ctrl Pts',(-71.499286106827,0.0221112224125953,
-101.882014068798));
#23836=CARTESIAN_POINT('Ctrl Pts',(-71.4993743526924,0.0221324119478113,
-101.882262612083));
#23837=CARTESIAN_POINT('Ctrl Pts',(-71.4994623109528,0.0221535482716482,
-101.882510352875));
#23838=CARTESIAN_POINT('Ctrl Pts',(-71.4995502644831,0.0221746992050154,
-101.882758090412));
#23839=CARTESIAN_POINT('Ctrl Pts',(-71.1249754475493,0.000402961545106217,
-102.019536869093));
#23840=CARTESIAN_POINT('Ctrl Pts',(-71.2498337198606,0.00766020743174241,
-101.973943942866));
#23841=CARTESIAN_POINT('Ctrl Pts',(-71.3746919921718,0.0149174533183786,
-101.928351016639));
#23842=CARTESIAN_POINT('Ctrl Pts',(-71.4995502644831,0.0221746992050148,
-101.882758090412));
#23843=CARTESIAN_POINT('',(-71.2060418705155,2.08166817117217E-16,-101.658452405258));
#23844=CARTESIAN_POINT('Ctrl Pts',(-71.124975960152,5.93046172723723,-107.949597022186));
#23845=CARTESIAN_POINT('Ctrl Pts',(-71.124444531672,5.93191700651268,-107.949613889587));
#23846=CARTESIAN_POINT('Ctrl Pts',(-71.1227720449596,5.93649691589196,-107.949672423109));
#23847=CARTESIAN_POINT('Ctrl Pts',(-71.115838041679,5.95548564468742,-107.949843257531));
#23848=CARTESIAN_POINT('Ctrl Pts',(-71.1102273169597,5.9708512545232,-107.949940211793));
#23849=CARTESIAN_POINT('Ctrl Pts',(-71.1041792426941,5.98741475677251,-107.949992161925));
#23850=CARTESIAN_POINT('Ctrl Pts',(-71.1006141582992,5.99717816092017,-107.950000273964));
#23851=CARTESIAN_POINT('Ctrl Pts',(-71.0999380484668,5.99902972241609,-107.95));
#23852=CARTESIAN_POINT('Ctrl Pts',(-71.099583741031,6.,-107.95));
#23853=CARTESIAN_POINT('Ctrl Pts',(-71.2498342285872,5.97605465101008,-107.942339741564));
#23854=CARTESIAN_POINT('Ctrl Pts',(-71.2481873471739,5.98062783599466,-107.942427298381));
#23855=CARTESIAN_POINT('Ctrl Pts',(-71.2417324406356,5.99844615137056,-107.943108609764));
#23856=CARTESIAN_POINT('Ctrl Pts',(-71.222688824581,6.05087242688524,-107.945030768774));
#23857=CARTESIAN_POINT('Ctrl Pts',(-71.202735966263,6.10580570763075,-107.947239708195));
#23858=CARTESIAN_POINT('Ctrl Pts',(-71.1852990888268,6.15377914453737,-107.948897246887));
#23859=CARTESIAN_POINT('Ctrl Pts',(-71.1746380484977,6.18311667273553,-107.949788229765));
#23860=CARTESIAN_POINT('Ctrl Pts',(-71.1716639991639,6.19131037031831,-107.95));
#23861=CARTESIAN_POINT('Ctrl Pts',(-71.170555827354,6.19436506316152,-107.95));
#23862=CARTESIAN_POINT('Ctrl Pts',(-71.3746924970224,6.02164757478294,-107.935082460943));
#23863=CARTESIAN_POINT('Ctrl Pts',(-71.3719373951989,6.02935581973102,-107.935472908878));
#23864=CARTESIAN_POINT('Ctrl Pts',(-71.3643778675314,6.05012165429468,-107.937512017716));
#23865=CARTESIAN_POINT('Ctrl Pts',(-71.3248781549867,6.157496923129,-107.942615263001));
#23866=CARTESIAN_POINT('Ctrl Pts',(-71.2979681803164,6.23187200229262,-107.946862365475));
#23867=CARTESIAN_POINT('Ctrl Pts',(-71.2648781488486,6.32329497724259,-107.948969720755));
#23868=CARTESIAN_POINT('Ctrl Pts',(-71.2459643513634,6.37616378464998,-107.949591702617));
#23869=CARTESIAN_POINT('Ctrl Pts',(-71.243389949861,6.38359101822054,-107.95));
#23870=CARTESIAN_POINT('Ctrl Pts',(-71.241527913677,6.38873012632304,-107.95));
#23871=CARTESIAN_POINT('Ctrl Pts',(-71.4995507654576,6.06724049855579,-107.927825180321));
#23872=CARTESIAN_POINT('Ctrl Pts',(-71.4957111858325,6.07805539364223,-107.9287485193));
#23873=CARTESIAN_POINT('Ctrl Pts',(-71.48371889734,6.1120489170111,-107.931938553361));
#23874=CARTESIAN_POINT('Ctrl Pts',(-71.4332019511036,6.25285912913773,-107.941309176545));
#23875=CARTESIAN_POINT('Ctrl Pts',(-71.3916442015717,6.36680923016425,-107.94669310563));
#23876=CARTESIAN_POINT('Ctrl Pts',(-71.3466221207365,6.48965178583955,-107.949568361152));
#23877=CARTESIAN_POINT('Ctrl Pts',(-71.3201199739812,6.56210068942826,-107.950014973511));
#23878=CARTESIAN_POINT('Ctrl Pts',(-71.3151159005581,6.57587166612277,-107.95));
#23879=CARTESIAN_POINT('Ctrl Pts',(-71.3125,6.58309518948457,-107.95));
#23880=CARTESIAN_POINT('',(-71.4995507654576,6.06724049855579,-107.927825180321));
#23881=CARTESIAN_POINT('Ctrl Pts',(-71.4995507654576,6.06724049855579,-107.927825180321));
#23882=CARTESIAN_POINT('Ctrl Pts',(-71.3746924970224,6.02164757478294,-107.935082460943));
#23883=CARTESIAN_POINT('Ctrl Pts',(-71.2498342285872,5.97605465101008,-107.942339741564));
#23884=CARTESIAN_POINT('Ctrl Pts',(-71.124975960152,5.93046172723723,-107.949597022186));
#23885=CARTESIAN_POINT('Ctrl Pts',(-71.4995507654576,6.0672404985558,-107.927825180321));
#23886=CARTESIAN_POINT('Ctrl Pts',(-71.4990207966871,6.06873325484982,-107.927952626779));
#23887=CARTESIAN_POINT('Ctrl Pts',(-71.4984892441742,6.07023015200047,-107.928079922666));
#23888=CARTESIAN_POINT('Ctrl Pts',(-71.497901536632,6.07188520349622,-107.928219936917));
#23889=CARTESIAN_POINT('Ctrl Pts',(-71.4972864948831,6.0736172312366,-107.928366463213));
#23890=CARTESIAN_POINT('Ctrl Pts',(-71.4966099619257,6.07552244369565,-107.928526920857));
#23891=CARTESIAN_POINT('Ctrl Pts',(-71.4958284703338,6.07772300303647,-107.928710903972));
#23892=CARTESIAN_POINT('Ctrl Pts',(-71.4950181155607,6.08000483662722,-107.928901682219));
#23893=CARTESIAN_POINT('Ctrl Pts',(-71.494094973154,6.08260404766213,-107.929117745108));
#23894=CARTESIAN_POINT('Ctrl Pts',(-71.4930300024624,6.08560145625756,-107.929364432221));
#23895=CARTESIAN_POINT('Ctrl Pts',(-71.491916951697,6.08873418841456,-107.92962225648));
#23896=CARTESIAN_POINT('Ctrl Pts',(-71.4906490574284,6.09230165151849,-107.929913509125));
#23897=CARTESIAN_POINT('Ctrl Pts',(-71.4892128900655,6.09633987574117,-107.930238780429));
#23898=CARTESIAN_POINT('Ctrl Pts',(-71.4876934020539,6.10061238147606,-107.930582922664));
#23899=CARTESIAN_POINT('Ctrl Pts',(-71.485985649468,6.10541155145357,-107.930965095528));
#23900=CARTESIAN_POINT('Ctrl Pts',(-71.4840939752819,6.11072251269302,-107.931380513992));
#23901=CARTESIAN_POINT('Ctrl Pts',(-71.4820490674957,6.11646368422841,-107.931829583108));
#23902=CARTESIAN_POINT('Ctrl Pts',(-71.4797893739799,6.12280247841059,-107.932317405233));
#23903=CARTESIAN_POINT('Ctrl Pts',(-71.4773416170346,6.12966027906724,-107.932832831001));
#23904=CARTESIAN_POINT('Ctrl Pts',(-71.474565129715,6.13743907287268,-107.933417477737));
#23905=CARTESIAN_POINT('Ctrl Pts',(-71.4715469228454,6.14588483863557,-107.93403743716));
#23906=CARTESIAN_POINT('Ctrl Pts',(-71.4683495425667,6.15481772739554,-107.934672492242));
#23907=CARTESIAN_POINT('Ctrl Pts',(-71.4633966290024,6.16865525125939,-107.93565622663));
#23908=CARTESIAN_POINT('Ctrl Pts',(-71.4580152424454,6.18365673275706,-107.936674546861));
#23909=CARTESIAN_POINT('Ctrl Pts',(-71.4524868534505,6.19902659477151,-107.937657083293));
#23910=CARTESIAN_POINT('Ctrl Pts',(-71.448955208538,6.20884516850782,-107.938284747119));
#23911=CARTESIAN_POINT('Ctrl Pts',(-71.4453646966192,6.21881124737631,-107.938898064687));
#23912=CARTESIAN_POINT('Ctrl Pts',(-71.4417814339702,6.22874060650452,-107.939484838886));
#23913=CARTESIAN_POINT('Ctrl Pts',(-71.4384221252368,6.23804938068721,-107.940034939697));
#23914=CARTESIAN_POINT('Ctrl Pts',(-71.4350697033288,6.24732450793948,-107.940561734482));
#23915=CARTESIAN_POINT('Ctrl Pts',(-71.4317622037675,6.25646134033559,-107.94106038123));
#23916=CARTESIAN_POINT('Ctrl Pts',(-71.4288719727465,6.26444548543854,-107.94149611955));
#23917=CARTESIAN_POINT('Ctrl Pts',(-71.4260160642607,6.27232401612069,-107.94191045257));
#23918=CARTESIAN_POINT('Ctrl Pts',(-71.4232040612964,6.2800714697516,-107.94230335782));
#23919=CARTESIAN_POINT('Ctrl Pts',(-71.4205610724397,6.287353266348,-107.942672647685));
#23920=CARTESIAN_POINT('Ctrl Pts',(-71.41795696231,6.29451903346519,-107.943023052383));
#23921=CARTESIAN_POINT('Ctrl Pts',(-71.4153838008589,6.30159180694595,-107.94335674417));
#23922=CARTESIAN_POINT('Ctrl Pts',(-71.4129144260191,6.30837930520969,-107.943676976741));
#23923=CARTESIAN_POINT('Ctrl Pts',(-71.4104736445188,6.31508092194651,-107.94398185317));
#23924=CARTESIAN_POINT('Ctrl Pts',(-71.4080380021628,6.32176249687741,-107.944274820287));
#23925=CARTESIAN_POINT('Ctrl Pts',(-71.4055526579071,6.32858041652497,-107.944573765714));
#23926=CARTESIAN_POINT('Ctrl Pts',(-71.4030698766341,6.33538518866313,-107.944860667827));
#23927=CARTESIAN_POINT('Ctrl Pts',(-71.4005586089811,6.34226352759248,-107.94513878121));
#23928=CARTESIAN_POINT('Ctrl Pts',(-71.3979671505498,6.34936150832369,-107.945425775418));
#23929=CARTESIAN_POINT('Ctrl Pts',(-71.3953454196391,6.35653763787639,-107.94570334598));
#23930=CARTESIAN_POINT('Ctrl Pts',(-71.392679664026,6.36383079184782,-107.94597187229));
#23931=CARTESIAN_POINT('Ctrl Pts',(-71.389865770012,6.37152923284606,-107.946255320844));
#23932=CARTESIAN_POINT('Ctrl Pts',(-71.3870029298745,6.37935775149941,-107.946528613934));
#23933=CARTESIAN_POINT('Ctrl Pts',(-71.3840958451337,6.38730453409799,-107.94678983111));
#23934=CARTESIAN_POINT('Ctrl Pts',(-71.3809670058234,6.39585750313803,-107.947070974124));
#23935=CARTESIAN_POINT('Ctrl Pts',(-71.3777870727492,6.40454701494908,-107.947338023315));
#23936=CARTESIAN_POINT('Ctrl Pts',(-71.3745834640428,6.41329921114333,-107.947587389251));
#23937=CARTESIAN_POINT('Ctrl Pts',(-71.3709749516525,6.4231575962656,-107.947868272515));
#23938=CARTESIAN_POINT('Ctrl Pts',(-71.3673366767398,6.43309474441533,-107.948126551975));
#23939=CARTESIAN_POINT('Ctrl Pts',(-71.3637310492388,6.44294166047392,-107.948357926994));
#23940=CARTESIAN_POINT('Ctrl Pts',(-71.3569401818035,6.46148742028461,-107.948793700539));
#23941=CARTESIAN_POINT('Ctrl Pts',(-71.3502675206052,6.4797066881043,-107.949130963775));
#23942=CARTESIAN_POINT('Ctrl Pts',(-71.3442156430593,6.4962365102952,-107.949371076525));
#23943=CARTESIAN_POINT('Ctrl Pts',(-71.3411205088944,6.50469041852693,-107.949493878279));
#23944=CARTESIAN_POINT('Ctrl Pts',(-71.3381883496994,6.51270076910323,-107.949592066599));
#23945=CARTESIAN_POINT('Ctrl Pts',(-71.3354757487876,6.52011387105198,-107.949670003794));
#23946=CARTESIAN_POINT('Ctrl Pts',(-71.3330312445731,6.52679430785273,-107.949740238159));
#23947=CARTESIAN_POINT('Ctrl Pts',(-71.3307652756209,6.53298908287031,-107.949794115064));
#23948=CARTESIAN_POINT('Ctrl Pts',(-71.328704925758,6.53862447881893,-107.949835858399));
#23949=CARTESIAN_POINT('Ctrl Pts',(-71.3267779835042,6.54389498300138,-107.949874898855));
#23950=CARTESIAN_POINT('Ctrl Pts',(-71.3250310441515,6.54867578942307,-107.949903374666));
#23951=CARTESIAN_POINT('Ctrl Pts',(-71.3234704637356,6.55294946252823,-107.949924777042));
#23952=CARTESIAN_POINT('Ctrl Pts',(-71.3220188858989,6.55692463041912,-107.949944684516));
#23953=CARTESIAN_POINT('Ctrl Pts',(-71.3207285830242,6.56046091966393,-107.949958491691));
#23954=CARTESIAN_POINT('Ctrl Pts',(-71.3195893262722,6.5635860256247,-107.949968587791));
#23955=CARTESIAN_POINT('Ctrl Pts',(-71.3184846160707,6.56661636661592,-107.94997837774));
#23956=CARTESIAN_POINT('Ctrl Pts',(-71.3175220329967,6.56925979976205,-107.949984684072));
#23957=CARTESIAN_POINT('Ctrl Pts',(-71.3166761339984,6.57158547788221,-107.949989099866));
#23958=CARTESIAN_POINT('Ctrl Pts',(-71.3158524584211,6.5738500558898,-107.949993399649));
#23959=CARTESIAN_POINT('Ctrl Pts',(-71.3151395029723,6.57581311704178,-107.949995903734));
#23960=CARTESIAN_POINT('Ctrl Pts',(-71.3144968795581,6.57758458484338,-107.949997507791));
#23961=CARTESIAN_POINT('Ctrl Pts',(-71.3138743484462,6.5793006658261,-107.949999061696));
#23962=CARTESIAN_POINT('Ctrl Pts',(-71.3133178685153,6.58083681331819,-107.949999767001));
#23963=CARTESIAN_POINT('Ctrl Pts',(-71.3127737075818,6.58233938722563,-107.949999953178));
#23964=CARTESIAN_POINT('Ctrl Pts',(-71.3126822667415,6.58259187984734,-107.949999984463));
#23965=CARTESIAN_POINT('Ctrl Pts',(-71.3125911327406,6.58284353638613,-107.95));
#23966=CARTESIAN_POINT('Ctrl Pts',(-71.3125,6.58309518948457,-107.95));
#23967=CARTESIAN_POINT('Ctrl Pts',(-71.4995507654576,6.06724049855579,-107.927825180321));
#23968=CARTESIAN_POINT('Ctrl Pts',(-71.8031162620164,5.21219142607177,-107.854823997106));
#23969=CARTESIAN_POINT('Ctrl Pts',(-72.1125000002033,4.23816712577613,-107.560861613326));
#23970=CARTESIAN_POINT('Ctrl Pts',(-72.1125,3.42868316199158,-107.149999999604));
#23971=CARTESIAN_POINT('Ctrl Pts',(-71.3746924970224,6.02164757478294,-107.935082460943));
#23972=CARTESIAN_POINT('Ctrl Pts',(-71.6811438088394,5.16661471749831,-107.883111714002));
#23973=CARTESIAN_POINT('Ctrl Pts',(-72.0098408305469,4.19555805202373,-107.611458539987));
#23974=CARTESIAN_POINT('Ctrl Pts',(-72.0395269177012,3.39266652940126,-107.206172926527));
#23975=CARTESIAN_POINT('Ctrl Pts',(-71.2498342285872,5.97605465101008,-107.942339741564));
#23976=CARTESIAN_POINT('Ctrl Pts',(-71.5591713556625,5.12103800892486,-107.911399430897));
#23977=CARTESIAN_POINT('Ctrl Pts',(-71.9071816608906,4.15294897827133,-107.662055466649));
#23978=CARTESIAN_POINT('Ctrl Pts',(-71.9665538354024,3.35664989681094,-107.262345853449));
#23979=CARTESIAN_POINT('Ctrl Pts',(-71.124975960152,5.93046172723723,-107.949597022186));
#23980=CARTESIAN_POINT('Ctrl Pts',(-71.4371989024855,5.0754613003514,-107.939687147793));
#23981=CARTESIAN_POINT('Ctrl Pts',(-71.8045224912342,4.11033990451893,-107.71265239331));
#23982=CARTESIAN_POINT('Ctrl Pts',(-71.8935807531036,3.32063326422062,-107.318518780371));
#23983=CARTESIAN_POINT('',(-72.1125,3.42868316190273,-107.14999999978));
#23984=CARTESIAN_POINT('',(-71.8935807531036,3.32063326422075,-107.318518780371));
#23985=CARTESIAN_POINT('Ctrl Pts',(-72.1125,3.42868316199158,-107.149999999604));
#23986=CARTESIAN_POINT('Ctrl Pts',(-72.1125000002033,4.23816712577613,-107.560861613326));
#23987=CARTESIAN_POINT('Ctrl Pts',(-71.8031162620164,5.21219142607177,-107.854823997106));
#23988=CARTESIAN_POINT('Ctrl Pts',(-71.4995507654576,6.06724049855579,-107.927825180321));
#23989=CARTESIAN_POINT('Origin',(-72.0125,6.00000000000001,-101.95));
#23990=CARTESIAN_POINT('',(-72.1125,0.97333333333333,-104.843548379105));
#23991=CARTESIAN_POINT('',(-71.9125,0.800000000000001,-104.943325909419));
#23992=CARTESIAN_POINT('',(-72.1125,3.10645162089483,-106.976666666667));
#23993=CARTESIAN_POINT('Origin',(-72.1125,6.00000000000001,-101.95));
#23994=CARTESIAN_POINT('',(-72.1125,3.10645162089483,-106.976666666667));
#23995=CARTESIAN_POINT('Ctrl Pts',(-72.1125,3.4286831619917,-107.149999999604));
#23996=CARTESIAN_POINT('Ctrl Pts',(-72.1125,3.31801931336453,-107.093831465749));
#23997=CARTESIAN_POINT('Ctrl Pts',(-72.1125,3.21069598181733,-107.036673848678));
#23998=CARTESIAN_POINT('Ctrl Pts',(-72.1125,3.10645162089484,-106.976666666667));
#23999=CARTESIAN_POINT('Ctrl Pts',(-72.0395269177012,3.39266652940138,-107.206172926527));
#24000=CARTESIAN_POINT('Ctrl Pts',(-72.0435852768747,3.28290392767118,-107.150766682816));
#24001=CARTESIAN_POINT('Ctrl Pts',(-72.0458333333333,3.1763983554736,-107.093853853762));
#24002=CARTESIAN_POINT('Ctrl Pts',(-72.0458333333333,3.07319244412351,-107.034444444444));
#24003=CARTESIAN_POINT('Ctrl Pts',(-71.9665538354024,3.35664989681107,-107.262345853449));
#24004=CARTESIAN_POINT('Ctrl Pts',(-71.9746705537493,3.24778854197784,-107.207701899883));
#24005=CARTESIAN_POINT('Ctrl Pts',(-71.9791666666667,3.14210072912987,-107.151033858845));
#24006=CARTESIAN_POINT('Ctrl Pts',(-71.9791666666667,3.03993326735219,-107.092222222222));
#24007=CARTESIAN_POINT('Ctrl Pts',(-71.8935807531036,3.32063326422075,-107.318518780371));
#24008=CARTESIAN_POINT('Ctrl Pts',(-71.905755830624,3.2126731562845,-107.26463711695));
#24009=CARTESIAN_POINT('Ctrl Pts',(-71.9125,3.10780310278613,-107.208213863928));
#24010=CARTESIAN_POINT('Ctrl Pts',(-71.9125,3.00667409058086,-107.15));
#24011=CARTESIAN_POINT('Ctrl Pts',(-72.1125,3.10645162089484,-106.976666666667));
#24012=CARTESIAN_POINT('Ctrl Pts',(-72.1125,3.21069598181733,-107.036673848678));
#24013=CARTESIAN_POINT('Ctrl Pts',(-72.1125,3.31801931336453,-107.093831465749));
#24014=CARTESIAN_POINT('Ctrl Pts',(-72.1125,3.4286831619917,-107.149999999604));
#24015=CARTESIAN_POINT('Ctrl Pts',(-72.1125,0.800000000395794,-104.521316838008));
#24016=CARTESIAN_POINT('Ctrl Pts',(-72.1125000002033,0.389138161249151,
-103.71183243009));
#24017=CARTESIAN_POINT('Ctrl Pts',(-71.8031182842413,0.0951762823709496,
-102.737814086272));
#24018=CARTESIAN_POINT('Ctrl Pts',(-71.4995502644836,0.022174699205149,
-101.882758090414));
#24019=CARTESIAN_POINT('Ctrl Pts',(-72.0395269177012,0.74382707347345,-104.557333470599));
#24020=CARTESIAN_POINT('Ctrl Pts',(-72.0098408142592,0.338541237647051,
-103.754441507459));
#24021=CARTESIAN_POINT('Ctrl Pts',(-71.6811442271336,0.0668883759257339,
-102.783386394673));
#24022=CARTESIAN_POINT('Ctrl Pts',(-71.374691992172,0.0149174533184618,
-101.92835101664));
#24023=CARTESIAN_POINT('Ctrl Pts',(-71.9665538354024,0.687654146551105,
-104.593350103189));
#24024=CARTESIAN_POINT('Ctrl Pts',(-71.9071816283152,0.287944314044952,
-103.797050584828));
#24025=CARTESIAN_POINT('Ctrl Pts',(-71.5591701700259,0.0386004694805184,
-102.828958703074));
#24026=CARTESIAN_POINT('Ctrl Pts',(-71.2498337198604,0.00766020743177456,
-101.973943942866));
#24027=CARTESIAN_POINT('Ctrl Pts',(-71.8935807531036,0.63148121962876,-104.629366735779));
#24028=CARTESIAN_POINT('Ctrl Pts',(-71.8045224423712,0.237347390442852,
-103.839659662198));
#24029=CARTESIAN_POINT('Ctrl Pts',(-71.4371961129181,0.0103125630353027,
-102.874531011475));
#24030=CARTESIAN_POINT('Ctrl Pts',(-71.1249754475488,0.000402961545087344,
-102.019536869091));
#24031=CARTESIAN_POINT('',(-72.1125,0.800000000220446,-104.521316838097));
#24032=CARTESIAN_POINT('Ctrl Pts',(-71.4995502644836,0.022174699205149,
-101.882758090414));
#24033=CARTESIAN_POINT('Ctrl Pts',(-71.8031182842413,0.0951762823709496,
-102.737814086272));
#24034=CARTESIAN_POINT('Ctrl Pts',(-72.1125000002033,0.389138161249151,
-103.71183243009));
#24035=CARTESIAN_POINT('Ctrl Pts',(-72.1125,0.800000000395794,-104.521316838008));
#24036=CARTESIAN_POINT('',(-72.1125,0.800000000220446,-104.521316838097));
#24037=CARTESIAN_POINT('Ctrl Pts',(-72.1125,0.973333333333336,-104.843548379105));
#24038=CARTESIAN_POINT('Ctrl Pts',(-72.1125,0.913326151321781,-104.739304018183));
#24039=CARTESIAN_POINT('Ctrl Pts',(-72.1125,0.856168534250963,-104.631980686636));
#24040=CARTESIAN_POINT('Ctrl Pts',(-72.1125,0.800000000395737,-104.521316838008));
#24041=CARTESIAN_POINT('Ctrl Pts',(-72.0458333333333,0.915555555555558,
-104.876807555876));
#24042=CARTESIAN_POINT('Ctrl Pts',(-72.0458333333333,0.856146146238371,
-104.773601644526));
#24043=CARTESIAN_POINT('Ctrl Pts',(-72.0435852768747,0.799233317184014,
-104.667096072329));
#24044=CARTESIAN_POINT('Ctrl Pts',(-72.0395269177012,0.743827073473394,
-104.557333470599));
#24045=CARTESIAN_POINT('Ctrl Pts',(-71.9791666666667,0.85777777777778,-104.910066732648));
#24046=CARTESIAN_POINT('Ctrl Pts',(-71.9791666666667,0.798966141154961,
-104.80789927087));
#24047=CARTESIAN_POINT('Ctrl Pts',(-71.9746705537493,0.742298100117066,
-104.702211458022));
#24048=CARTESIAN_POINT('Ctrl Pts',(-71.9665538354024,0.68765414655105,-104.593350103189));
#24049=CARTESIAN_POINT('Ctrl Pts',(-71.9125,0.800000000000002,-104.943325909419));
#24050=CARTESIAN_POINT('Ctrl Pts',(-71.9125,0.741786136071551,-104.842196897214));
#24051=CARTESIAN_POINT('Ctrl Pts',(-71.905755830624,0.685362883050117,-104.737326843716));
#24052=CARTESIAN_POINT('Ctrl Pts',(-71.8935807531036,0.631481219628707,
-104.629366735779));
#24053=CARTESIAN_POINT('Ctrl Pts',(-72.1125,0.800000000395737,-104.521316838008));
#24054=CARTESIAN_POINT('Ctrl Pts',(-72.1125,0.856168534250963,-104.631980686636));
#24055=CARTESIAN_POINT('Ctrl Pts',(-72.1125,0.913326151321781,-104.739304018183));
#24056=CARTESIAN_POINT('Ctrl Pts',(-72.1125,0.973333333333336,-104.843548379105));
#24057=CARTESIAN_POINT('Origin',(-71.3125,0.800000000000001,-66.85));
#24058=CARTESIAN_POINT('',(-71.3125,5.55111512312578E-16,37.8669048105155));
#24059=CARTESIAN_POINT('',(-71.3125,0.,-66.85));
#24060=CARTESIAN_POINT('',(-71.4995507644729,0.0221748194419996,38.3827594987134));
#24061=CARTESIAN_POINT('Ctrl Pts',(-71.4995507644729,0.0221748194419995,
38.3827594987134));
#24062=CARTESIAN_POINT('Ctrl Pts',(-71.4990207956831,0.0220473729800413,
38.3812667424329));
#24063=CARTESIAN_POINT('Ctrl Pts',(-71.4984892431503,0.0219200770893842,
38.3797698452961));
#24064=CARTESIAN_POINT('Ctrl Pts',(-71.4979015355679,0.021780062829885,
38.378114793822));
#24065=CARTESIAN_POINT('Ctrl Pts',(-71.4972864937771,0.0216335365241201,
38.3763827661041));
#24066=CARTESIAN_POINT('Ctrl Pts',(-71.4966099607556,0.021473078866498,
38.3744775536761));
#24067=CARTESIAN_POINT('Ctrl Pts',(-71.4958284690637,0.0212890957288703,
38.3722769943803));
#24068=CARTESIAN_POINT('Ctrl Pts',(-71.4950181141868,0.02109831745909,38.3699951608361));
#24069=CARTESIAN_POINT('Ctrl Pts',(-71.4940949716375,0.0208822545381878,
38.3673959498629));
#24070=CARTESIAN_POINT('Ctrl Pts',(-71.4930300007572,0.0206355673841659,
38.3643985413472));
#24071=CARTESIAN_POINT('Ctrl Pts',(-71.4919169497944,0.0203777430817619,
38.3612658092734));
#24072=CARTESIAN_POINT('Ctrl Pts',(-71.4906490552782,0.0200864903833777,
38.3576983462725));
#24073=CARTESIAN_POINT('Ctrl Pts',(-71.4892128876169,0.0197612190168368,
38.3536601221728));
#24074=CARTESIAN_POINT('Ctrl Pts',(-71.4876933992894,0.0194170767150211,
38.349387616567));
#24075=CARTESIAN_POINT('Ctrl Pts',(-71.485985646331,0.0190349037745015,
38.3445884467408));
#24076=CARTESIAN_POINT('Ctrl Pts',(-71.4840939717242,0.0186194852263588,
38.3392774856718));
#24077=CARTESIAN_POINT('Ctrl Pts',(-71.4820490634828,0.0181704160208765,
38.33353631432));
#24078=CARTESIAN_POINT('Ctrl Pts',(-71.4797893694556,0.0176825937973,38.3271975203437));
#24079=CARTESIAN_POINT('Ctrl Pts',(-71.4773416119619,0.0171671679305936,
38.3203397199083));
#24080=CARTESIAN_POINT('Ctrl Pts',(-71.4745651240188,0.016582521082149,
38.3125609263497));
#24081=CARTESIAN_POINT('Ctrl Pts',(-71.4715469164779,0.0159625615450801,
38.3041151608526));
#24082=CARTESIAN_POINT('Ctrl Pts',(-71.4683495355182,0.0153275063577457,
38.295182272364));
#24083=CARTESIAN_POINT('Ctrl Pts',(-71.4633966211176,0.0143437718506017,
38.2813447495314));
#24084=CARTESIAN_POINT('Ctrl Pts',(-71.4580152337396,0.0133254515238729,
38.2663432691807));
#24085=CARTESIAN_POINT('Ctrl Pts',(-71.4524868440586,0.0123429150381997,
38.2509734082674));
#24086=CARTESIAN_POINT('Ctrl Pts',(-71.4489551985486,0.0117152511490301,
38.241154834792));
#24087=CARTESIAN_POINT('Ctrl Pts',(-71.4453646860824,0.0111019335359449,
38.2311887561521));
#24088=CARTESIAN_POINT('Ctrl Pts',(-71.4417814229731,0.010515159313331,
38.2212593972102));
#24089=CARTESIAN_POINT('Ctrl Pts',(-71.4384221138081,0.00996505847963049,
38.2119506232022));
#24090=CARTESIAN_POINT('Ctrl Pts',(-71.4350696915454,0.00943826368962347,
38.2026754960875));
#24091=CARTESIAN_POINT('Ctrl Pts',(-71.4317621917286,0.00893961695450685,
38.1935386637876));
#24092=CARTESIAN_POINT('Ctrl Pts',(-71.4288719604788,0.00850387864572192,
38.1855545187534));
#24093=CARTESIAN_POINT('Ctrl Pts',(-71.4260160518402,0.00808954564913643,
38.1776759881089));
#24094=CARTESIAN_POINT('Ctrl Pts',(-71.4232040488063,0.00769664043506357,
38.1699285344855));
#24095=CARTESIAN_POINT('Ctrl Pts',(-71.4205610599081,0.00732735060630408,
38.1626467379619));
#24096=CARTESIAN_POINT('Ctrl Pts',(-71.41795694981,0.00697694595537342,
38.1554809708886));
#24097=CARTESIAN_POINT('Ctrl Pts',(-71.4153837884622,0.00664325422186796,
38.1484081974271));
#24098=CARTESIAN_POINT('Ctrl Pts',(-71.4129144136961,0.00632302170046841,
38.1416206991121));
#24099=CARTESIAN_POINT('Ctrl Pts',(-71.4104736323363,0.00601814532745467,
38.1349190823032));
#24100=CARTESIAN_POINT('Ctrl Pts',(-71.4080379901782,0.00572517827095886,
38.1282375072849));
#24101=CARTESIAN_POINT('Ctrl Pts',(-71.4055526461237,0.0054262329067401,
38.1214195875458));
#24102=CARTESIAN_POINT('Ctrl Pts',(-71.4030698651113,0.00513933086078111,
38.1146148153011));
#24103=CARTESIAN_POINT('Ctrl Pts',(-71.4005585977608,0.00486121754727409,
38.1077364762525));
#24104=CARTESIAN_POINT('Ctrl Pts',(-71.3979671396617,0.0045742234131711,
38.1006384954532));
#24105=CARTESIAN_POINT('Ctrl Pts',(-71.3953454091284,0.00429665292678922,
38.0934623658199));
#24106=CARTESIAN_POINT('Ctrl Pts',(-71.392679653921,0.00402812669221708,
38.0861692117592));
#24107=CARTESIAN_POINT('Ctrl Pts',(-71.3898657603368,0.00374467821706666,
38.0784707706709));
#24108=CARTESIAN_POINT('Ctrl Pts',(-71.3870029206609,0.00347138520559411,
38.0706422519179));
#24109=CARTESIAN_POINT('Ctrl Pts',(-71.384095836396,0.00321016810531405,
38.0626954692138));
#24110=CARTESIAN_POINT('Ctrl Pts',(-71.3809669976009,0.00292902517211406,
38.0541425000684));
#24111=CARTESIAN_POINT('Ctrl Pts',(-71.3777870650587,0.00266197605738847,
38.0454529881455));
#24112=CARTESIAN_POINT('Ctrl Pts',(-71.3745834568822,0.00241261019148575,
38.036700791836));
#24113=CARTESIAN_POINT('Ctrl Pts',(-71.3709749451015,0.00213172700751753,
38.0268424066186));
#24114=CARTESIAN_POINT('Ctrl Pts',(-71.3673366707961,0.00187344761883645,
38.0169052583702));
#24115=CARTESIAN_POINT('Ctrl Pts',(-71.3637310438776,0.0016420726621369,
38.0070583422105));
#24116=CARTESIAN_POINT('Ctrl Pts',(-71.356940177458,0.00120629922819576,
37.9885125819873));
#24117=CARTESIAN_POINT('Ctrl Pts',(-71.3502675171857,0.000869036069561573,
37.9702933137546));
#24118=CARTESIAN_POINT('Ctrl Pts',(-71.3442156403977,0.000628923369027201,
37.9537634911982));
#24119=CARTESIAN_POINT('Ctrl Pts',(-71.3411205066207,0.000506121640610308,
37.9453095827801));
#24120=CARTESIAN_POINT('Ctrl Pts',(-71.3381883477706,0.000407933340316306,
37.9372992320297));
#24121=CARTESIAN_POINT('Ctrl Pts',(-71.3354757471578,0.000329996159329049,
37.9298861299241));
#24122=CARTESIAN_POINT('Ctrl Pts',(-71.3330312432178,0.000259761807429823,
37.9232056929958));
#24123=CARTESIAN_POINT('Ctrl Pts',(-71.330765274502,0.00020588491124297,
37.9170109178627));
#24124=CARTESIAN_POINT('Ctrl Pts',(-71.328704924838,0.000164141582166488,
37.9113755218124));
#24125=CARTESIAN_POINT('Ctrl Pts',(-71.3267779827721,0.0001251011327827,
37.9061050175396));
#24126=CARTESIAN_POINT('Ctrl Pts',(-71.3250310435743,9.66253253805291E-5,
37.9013242110388));
#24127=CARTESIAN_POINT('Ctrl Pts',(-71.3234704632832,7.52229519629388E-5,
37.8970505378663));
#24128=CARTESIAN_POINT('Ctrl Pts',(-71.3220188855637,5.53154799969384E-5,
37.8930753699158));
#24129=CARTESIAN_POINT('Ctrl Pts',(-71.3207285827801,4.15083061174377E-5,
37.889539080621));
#24130=CARTESIAN_POINT('Ctrl Pts',(-71.3195893260971,3.1412207024184E-5,
37.8864139746195));
#24131=CARTESIAN_POINT('Ctrl Pts',(-71.3184846159629,2.16222596392345E-5,
37.8833836335894));
#24132=CARTESIAN_POINT('Ctrl Pts',(-71.3175220329355,1.53159280140433E-5,
37.880740200413));
#24133=CARTESIAN_POINT('Ctrl Pts',(-71.3166761339687,1.09001335865111E-5,
37.8784145222705));
#24134=CARTESIAN_POINT('Ctrl Pts',(-71.3158524584221,6.60035071474075E-6,
37.8761499442413));
#24135=CARTESIAN_POINT('Ctrl Pts',(-71.3151395029899,4.09626587467967E-6,
37.8741868830752));
#24136=CARTESIAN_POINT('Ctrl Pts',(-71.3144968795844,2.49220892911683E-6,
37.8724154152659));
#24137=CARTESIAN_POINT('Ctrl Pts',(-71.3138743484812,9.38304525135002E-7,
37.8706993342765));
#24138=CARTESIAN_POINT('Ctrl Pts',(-71.3133178685519,2.32998667997062E-7,
37.8691631867836));
#24139=CARTESIAN_POINT('Ctrl Pts',(-71.31277370762,4.68224151672914E-8,
37.8676606128799));
#24140=CARTESIAN_POINT('Ctrl Pts',(-71.3126822667669,1.55373405006649E-8,
37.8674081202228));
#24141=CARTESIAN_POINT('Ctrl Pts',(-71.3125911327533,5.5612328912237E-16,
37.867156463649));
#24142=CARTESIAN_POINT('Ctrl Pts',(-71.3125,5.55111512312578E-16,37.8669048105155));
#24143=CARTESIAN_POINT('',(-72.1125,0.800000000220445,41.0213168380973));
#24144=CARTESIAN_POINT('Ctrl Pts',(-72.1125,0.800000000395795,41.0213168380085));
#24145=CARTESIAN_POINT('Ctrl Pts',(-72.1125000002033,0.389138386673939,
40.2118328742239));
#24146=CARTESIAN_POINT('Ctrl Pts',(-71.8031180421414,0.095176430570246,
39.2378135490065));
#24147=CARTESIAN_POINT('Ctrl Pts',(-71.4995507644729,0.0221748194419993,
38.3827594987134));
#24148=CARTESIAN_POINT('',(-72.1125,0.800000000000001,-66.85));
#24149=CARTESIAN_POINT('Origin',(-67.35,0.,-101.95));
#24150=CARTESIAN_POINT('',(-68.15,0.,-66.85));
#24151=CARTESIAN_POINT('',(-71.099583741031,2.22044604925031E-15,38.45));
#24152=CARTESIAN_POINT('',(-67.35,2.22044604925031E-15,38.45));
#24153=CARTESIAN_POINT('',(-71.2060418705155,1.38777878078145E-15,38.1584524052577));
#24154=CARTESIAN_POINT('Ctrl Pts',(-71.4995502651826,6.06724190764745,44.4278253006268));
#24155=CARTESIAN_POINT('Ctrl Pts',(-71.4893114124994,6.09608154849019,44.4302875246095));
#24156=CARTESIAN_POINT('Ctrl Pts',(-71.3975276772687,6.35256309319244,44.4503655595348));
#24157=CARTESIAN_POINT('Ctrl Pts',(-71.3203476800974,6.56142467898143,44.45));
#24158=CARTESIAN_POINT('Ctrl Pts',(-71.3125,6.58309518948451,44.45));
#24159=CARTESIAN_POINT('Ctrl Pts',(-71.3746919924042,6.02164898271828,44.435082546577));
#24160=CARTESIAN_POINT('Ctrl Pts',(-71.3673450818445,6.04220422326533,44.4361237366707));
#24161=CARTESIAN_POINT('Ctrl Pts',(-71.3026150186436,6.22408187278844,44.4524101433031));
#24162=CARTESIAN_POINT('Ctrl Pts',(-71.2471140006817,6.37331286135218,44.45));
#24163=CARTESIAN_POINT('Ctrl Pts',(-71.241527913677,6.38873012632301,44.45));
#24164=CARTESIAN_POINT('Ctrl Pts',(-71.2498337196257,5.97605605778911,44.4423397925273));
#24165=CARTESIAN_POINT('Ctrl Pts',(-71.2454420638959,5.98825113903958,44.4425732724023));
#24166=CARTESIAN_POINT('Ctrl Pts',(-71.2057778485336,6.09746688787165,44.4476681728695));
#24167=CARTESIAN_POINT('Ctrl Pts',(-71.173880321266,6.18520104372293,44.45));
#24168=CARTESIAN_POINT('Ctrl Pts',(-71.170555827354,6.1943650631615,44.45));
#24169=CARTESIAN_POINT('Ctrl Pts',(-71.1249754468472,5.93046313285994,44.4495970384775));
#24170=CARTESIAN_POINT('Ctrl Pts',(-71.1235583328476,5.93434379913903,44.4496420163942));
#24171=CARTESIAN_POINT('Ctrl Pts',(-71.1109271247571,5.96893411817337,44.4500077127941));
#24172=CARTESIAN_POINT('Ctrl Pts',(-71.1006466418503,5.99708922609368,44.45));
#24173=CARTESIAN_POINT('Ctrl Pts',(-71.099583741031,6.,44.45));
#24174=CARTESIAN_POINT('',(-71.4995502651826,6.06724190764745,44.4278253006268));
#24175=CARTESIAN_POINT('Ctrl Pts',(-71.3125,6.58309518948451,44.45));
#24176=CARTESIAN_POINT('Ctrl Pts',(-71.3130414730319,6.58159997091307,44.45));
#24177=CARTESIAN_POINT('Ctrl Pts',(-71.3135844616982,6.58010061545634,44.4499994907131));
#24178=CARTESIAN_POINT('Ctrl Pts',(-71.3141854581767,6.57844322897758,44.4499982245172));
#24179=CARTESIAN_POINT('Ctrl Pts',(-71.3148143991277,6.57670877916745,44.4499968994472));
#24180=CARTESIAN_POINT('Ctrl Pts',(-71.3155068597438,6.57480128397541,44.449994750064));
#24181=CARTESIAN_POINT('Ctrl Pts',(-71.3163076849504,6.57259867099708,44.4499909384083));
#24182=CARTESIAN_POINT('Ctrl Pts',(-71.31713807453,6.57031474330561,44.4499869860361));
#24183=CARTESIAN_POINT('Ctrl Pts',(-71.3180849093956,6.56771369413082,44.4499812519661));
#24184=CARTESIAN_POINT('Ctrl Pts',(-71.3191778993281,6.56471475376676,44.4499721280523));
#24185=CARTESIAN_POINT('Ctrl Pts',(-71.3203202083267,6.5615804919933,44.4499625924395));
#24186=CARTESIAN_POINT('Ctrl Pts',(-71.3216220762682,6.55801185344091,44.4499493502156));
#24187=CARTESIAN_POINT('Ctrl Pts',(-71.3230967980082,6.55397281294346,44.4499298143412));
#24188=CARTESIAN_POINT('Ctrl Pts',(-71.3246570200264,6.54969960007501,44.449909145831));
#24189=CARTESIAN_POINT('Ctrl Pts',(-71.3264106108636,6.54490016320096,44.4498814075098));
#24190=CARTESIAN_POINT('Ctrl Pts',(-71.3283521807648,6.53958932246207,44.4498429273082));
#24191=CARTESIAN_POINT('Ctrl Pts',(-71.3304508793576,6.53384868238601,44.4498013329547));
#24192=CARTESIAN_POINT('Ctrl Pts',(-71.3327690552956,6.52751095521831,44.4497471254782));
#24193=CARTESIAN_POINT('Ctrl Pts',(-71.3352778810258,6.52065461386513,44.449675664339));
#24194=CARTESIAN_POINT('Ctrl Pts',(-71.3381228093806,6.51287974146511,44.4495946296865));
#24195=CARTESIAN_POINT('Ctrl Pts',(-71.3412126011462,6.50443878957283,44.4494912678601));
#24196=CARTESIAN_POINT('Ctrl Pts',(-71.3444812014443,6.49551117516062,44.4493604961181));
#24197=CARTESIAN_POINT('Ctrl Pts',(-71.3495556188186,6.48165128482434,44.4491574763729));
#24198=CARTESIAN_POINT('Ctrl Pts',(-71.3550592025856,6.46662336130317,44.4488871120809));
#24199=CARTESIAN_POINT('Ctrl Pts',(-71.3606972674011,6.45122664552515,44.4485468198015));
#24200=CARTESIAN_POINT('Ctrl Pts',(-71.3642934132123,6.44140610660548,44.4483297700344));
#24201=CARTESIAN_POINT('Ctrl Pts',(-71.3679432201769,6.43143836252666,44.4480847940351));
#24202=CARTESIAN_POINT('Ctrl Pts',(-71.3715786926663,6.42150762201508,44.4478155852532));
#24203=CARTESIAN_POINT('Ctrl Pts',(-71.3749869481252,6.41219755278548,44.4475632020201));
#24204=CARTESIAN_POINT('Ctrl Pts',(-71.3783821050343,6.40292137962196,44.4472896652331));
#24205=CARTESIAN_POINT('Ctrl Pts',(-71.3817254153414,6.39378372955202,44.4469992734443));
#24206=CARTESIAN_POINT('Ctrl Pts',(-71.3846464426477,6.38580022729881,44.4467455601284));
#24207=CARTESIAN_POINT('Ctrl Pts',(-71.387527894579,6.37792247617558,44.4464790726766));
#24208=CARTESIAN_POINT('Ctrl Pts',(-71.3903601144382,6.37017591351312,44.4462021116398));
#24209=CARTESIAN_POINT('Ctrl Pts',(-71.3930216639747,6.36289616077923,44.4459418403488));
#24210=CARTESIAN_POINT('Ctrl Pts',(-71.3956396564043,6.35573249576139,44.4456723848728));
#24211=CARTESIAN_POINT('Ctrl Pts',(-71.3982221077352,6.34866190828219,44.445394066011));
#24212=CARTESIAN_POINT('Ctrl Pts',(-71.4007009278315,6.34187505653155,44.4451269158115));
#24213=CARTESIAN_POINT('Ctrl Pts',(-71.4031469208213,6.3351742015686,44.4448516557739));
#24214=CARTESIAN_POINT('Ctrl Pts',(-71.4055836100285,6.32849354473077,44.4445661970812));
#24215=CARTESIAN_POINT('Ctrl Pts',(-71.4080709304171,6.32167407267327,44.4442748069341));
#24216=CARTESIAN_POINT('Ctrl Pts',(-71.4105513495158,6.31486792632762,44.4439724845748));
#24217=CARTESIAN_POINT('Ctrl Pts',(-71.4130558872244,6.30798832458474,44.4436551603464));
#24218=CARTESIAN_POINT('Ctrl Pts',(-71.4156402710321,6.30088939719107,44.4433277196396));
#24219=CARTESIAN_POINT('Ctrl Pts',(-71.4182502612752,6.29371244739847,44.4429842570855));
#24220=CARTESIAN_POINT('Ctrl Pts',(-71.4208995017854,6.28641857841381,44.4426219452));
#24221=CARTESIAN_POINT('Ctrl Pts',(-71.4236959667089,6.2787193722855,44.4422394988064));
#24222=CARTESIAN_POINT('Ctrl Pts',(-71.4265360438204,6.27089020577405,44.4418359995615));
#24223=CARTESIAN_POINT('Ctrl Pts',(-71.4294150367517,6.2629429051824,44.4414106861683));
#24224=CARTESIAN_POINT('Ctrl Pts',(-71.432513653979,6.2543893438808,44.4409529276955));
#24225=CARTESIAN_POINT('Ctrl Pts',(-71.4356571739941,6.24569938969948,44.4404698354042));
#24226=CARTESIAN_POINT('Ctrl Pts',(-71.4388186030689,6.23694695263107,44.4399643096487));
#24227=CARTESIAN_POINT('Ctrl Pts',(-71.4423797435989,6.22708791178466,44.4393948683567));
#24228=CARTESIAN_POINT('Ctrl Pts',(-71.4459633037202,6.21715035833354,44.4387968648388));
#24229=CARTESIAN_POINT('Ctrl Pts',(-71.449508394624,6.20730341158804,44.4381806263811));
#24230=CARTESIAN_POINT('Ctrl Pts',(-71.4561832905068,6.18876302825965,44.4370203380683));
#24231=CARTESIAN_POINT('Ctrl Pts',(-71.462718828944,6.17055030095169,44.4357930115265));
#24232=CARTESIAN_POINT('Ctrl Pts',(-71.4686322750488,6.15402777629251,44.4346162837261));
#24233=CARTESIAN_POINT('Ctrl Pts',(-71.4716575881422,6.14557486925647,44.4340142709641));
#24234=CARTESIAN_POINT('Ctrl Pts',(-71.4745196697734,6.13756600214882,44.4334264063996));
#24235=CARTESIAN_POINT('Ctrl Pts',(-71.4771650503419,6.13015493599191,44.4328699899702));
#24236=CARTESIAN_POINT('Ctrl Pts',(-71.4795488948579,6.12347656629865,44.4323685837568));
#24237=CARTESIAN_POINT('Ctrl Pts',(-71.4817565642925,6.1172842734726,44.4318928535763));
#24238=CARTESIAN_POINT('Ctrl Pts',(-71.4837629722623,6.11165176399895,44.4314531299649));
#24239=CARTESIAN_POINT('Ctrl Pts',(-71.48563944169,6.10638402583829,44.4310418836352));
#24240=CARTESIAN_POINT('Ctrl Pts',(-71.4873397401627,6.10160632696767,44.4306622124859));
#24241=CARTESIAN_POINT('Ctrl Pts',(-71.4888585907838,6.09733604160017,44.4303189395733));
#24242=CARTESIAN_POINT('Ctrl Pts',(-71.4902713563202,6.09336401702186,44.4299996427749));
#24243=CARTESIAN_POINT('Ctrl Pts',(-71.4915271008574,6.08983111529501,44.4297118654696));
#24244=CARTESIAN_POINT('Ctrl Pts',(-71.4926362835771,6.08670954431889,44.4294555274928));
#24245=CARTESIAN_POINT('Ctrl Pts',(-71.4937118264108,6.08368264601486,44.4292069638711));
#24246=CARTESIAN_POINT('Ctrl Pts',(-71.4946494646873,6.08104279063262,44.4289879910269));
#24247=CARTESIAN_POINT('Ctrl Pts',(-71.4954741515926,6.07872068925268,44.4287942346018));
#24248=CARTESIAN_POINT('Ctrl Pts',(-71.4962771694046,6.0764596023391,44.4286055692312));
#24249=CARTESIAN_POINT('Ctrl Pts',(-71.4969730091871,6.07450002927982,44.4284408297404));
#24250=CARTESIAN_POINT('Ctrl Pts',(-71.4976008840125,6.07273187234974,44.4282915024191));
#24251=CARTESIAN_POINT('Ctrl Pts',(-71.4982091353165,6.07101897717568,44.4281468421553));
#24252=CARTESIAN_POINT('Ctrl Pts',(-71.498753555852,6.06948585391535,44.4280166533539));
#24253=CARTESIAN_POINT('Ctrl Pts',(-71.4992861074866,6.06798592939874,44.427888777429));
#24254=CARTESIAN_POINT('Ctrl Pts',(-71.4993743533654,6.06773738606794,44.4278675878905));
#24255=CARTESIAN_POINT('Ctrl Pts',(-71.499462311639,6.06748964522966,44.4278464515634));
#24256=CARTESIAN_POINT('Ctrl Pts',(-71.4995502651826,6.06724190764745,44.4278253006268));
#24257=CARTESIAN_POINT('',(-71.1249754468472,5.93046313285994,44.4495970384775));
#24258=CARTESIAN_POINT('Ctrl Pts',(-71.1249754468472,5.93046313285994,44.4495970384775));
#24259=CARTESIAN_POINT('Ctrl Pts',(-71.2498337196257,5.97605605778911,44.4423397925273));
#24260=CARTESIAN_POINT('Ctrl Pts',(-71.3746919924042,6.02164898271828,44.435082546577));
#24261=CARTESIAN_POINT('Ctrl Pts',(-71.4995502651826,6.06724190764745,44.4278253006268));
#24262=CARTESIAN_POINT('Ctrl Pts',(-71.1249754468472,5.93046313285994,44.4495970384775));
#24263=CARTESIAN_POINT('Ctrl Pts',(-71.1248515871029,5.93080231399357,44.4496009696738));
#24264=CARTESIAN_POINT('Ctrl Pts',(-71.1247261187253,5.93114590045165,44.4496049290215));
#24265=CARTESIAN_POINT('Ctrl Pts',(-71.1245663839378,5.93158332280883,44.4496099171765));
#24266=CARTESIAN_POINT('Ctrl Pts',(-71.124399215446,5.93204110183689,44.4496151374692));
#24267=CARTESIAN_POINT('Ctrl Pts',(-71.1241946568714,5.93260127070091,44.4496214810533));
#24268=CARTESIAN_POINT('Ctrl Pts',(-71.1239352648988,5.93331159796484,44.4496293766394));
#24269=CARTESIAN_POINT('Ctrl Pts',(-71.1236418501879,5.9341150941825,44.4496383078375));
#24270=CARTESIAN_POINT('Ctrl Pts',(-71.1232782835419,5.93511069785848,44.4496492227469));
#24271=CARTESIAN_POINT('Ctrl Pts',(-71.1228435341425,5.93630123568408,44.4496618627573));
#24272=CARTESIAN_POINT('Ctrl Pts',(-71.1223678608009,5.93760384152227,44.4496756926004));
#24273=CARTESIAN_POINT('Ctrl Pts',(-71.1218074187549,5.93913858691462,44.4496915586601));
#24274=CARTESIAN_POINT('Ctrl Pts',(-71.1211844497222,5.94084456975602,44.4497083791692));
#24275=CARTESIAN_POINT('Ctrl Pts',(-71.1202527747972,5.94339593483545,44.4497335349083));
#24276=CARTESIAN_POINT('Ctrl Pts',(-71.1191829294765,5.94632569724299,44.4497606651809));
#24277=CARTESIAN_POINT('Ctrl Pts',(-71.1180892995269,5.94932062429705,44.4497859629222));
#24278=CARTESIAN_POINT('Ctrl Pts',(-71.1173517755765,5.95134034809186,44.4498030232543));
#24279=CARTESIAN_POINT('Ctrl Pts',(-71.1166045454595,5.95338666559846,44.4498192636616));
#24280=CARTESIAN_POINT('Ctrl Pts',(-71.1158742947463,5.95538649749497,44.4498341339902));
#24281=CARTESIAN_POINT('Ctrl Pts',(-71.1152379642737,5.95712912362704,44.449847091791));
#24282=CARTESIAN_POINT('Ctrl Pts',(-71.1146147683738,5.95883579007516,44.4498590203309));
#24283=CARTESIAN_POINT('Ctrl Pts',(-71.114008582509,5.9604958820991,44.4498699506463));
#24284=CARTESIAN_POINT('Ctrl Pts',(-71.1134416131077,5.96204857647174,44.4498801738382));
#24285=CARTESIAN_POINT('Ctrl Pts',(-71.1128897129432,5.96356001028047,44.4498895316588));
#24286=CARTESIAN_POINT('Ctrl Pts',(-71.1123401813906,5.96506496295198,44.4498982944035));
#24287=CARTESIAN_POINT('Ctrl Pts',(-71.1117897476999,5.96657238622816,44.4499070715337));
#24288=CARTESIAN_POINT('Ctrl Pts',(-71.1112385931528,5.96808178899618,44.4499153019222));
#24289=CARTESIAN_POINT('Ctrl Pts',(-71.1106726306169,5.96963174796688,44.4499231469468));
#24290=CARTESIAN_POINT('Ctrl Pts',(-71.1100599015201,5.97130978299583,44.4499316402207));
#24291=CARTESIAN_POINT('Ctrl Pts',(-71.1094299980603,5.97303485537856,44.4499396657415));
#24292=CARTESIAN_POINT('Ctrl Pts',(-71.1087859002502,5.97479880212128,44.4499470747354));
#24293=CARTESIAN_POINT('Ctrl Pts',(-71.1080330495214,5.97686058306483,44.4499557347034));
#24294=CARTESIAN_POINT('Ctrl Pts',(-71.1072611033227,5.97897466126154,44.4499635242262));
#24295=CARTESIAN_POINT('Ctrl Pts',(-71.10649893061,5.98106197314173,44.4499701125205));
#24296=CARTESIAN_POINT('Ctrl Pts',(-71.1055840057745,5.98356761713372,44.4499780212187));
#24297=CARTESIAN_POINT('Ctrl Pts',(-71.1046847838885,5.98603025599151,44.4499841533453));
#24298=CARTESIAN_POINT('Ctrl Pts',(-71.1038687720391,5.98826500948254,44.4499885241555));
#24299=CARTESIAN_POINT('Ctrl Pts',(-71.1032398030133,5.98998752212432,44.4499918931068));
#24300=CARTESIAN_POINT('Ctrl Pts',(-71.1026610568414,5.99157249064109,44.4499942405047));
#24301=CARTESIAN_POINT('Ctrl Pts',(-71.1021565447218,5.99295415655121,44.4499958630061));
#24302=CARTESIAN_POINT('Ctrl Pts',(-71.101698261038,5.99420922044048,44.4499973368377));
#24303=CARTESIAN_POINT('Ctrl Pts',(-71.1013015496871,5.99529565802496,44.4499982237945));
#24304=CARTESIAN_POINT('Ctrl Pts',(-71.1009716247545,5.99619919007953,44.4499987961535));
#24305=CARTESIAN_POINT('Ctrl Pts',(-71.1006620428143,5.99704701083741,44.4499993332212));
#24306=CARTESIAN_POINT('Ctrl Pts',(-71.1004114664506,5.9977332351973,44.4499995974697));
#24307=CARTESIAN_POINT('Ctrl Pts',(-71.1002088601892,5.99828808589258,44.4499997557792));
#24308=CARTESIAN_POINT('Ctrl Pts',(-71.1000192696623,5.99880729213499,44.4499999039186));
#24309=CARTESIAN_POINT('Ctrl Pts',(-71.0998717695326,5.99921122722298,44.4499999587511));
#24310=CARTESIAN_POINT('Ctrl Pts',(-71.0997415471272,5.99956784464617,44.4499999844368));
#24311=CARTESIAN_POINT('Ctrl Pts',(-71.0996870475666,5.99971709310149,44.4499999951866));
#24312=CARTESIAN_POINT('Ctrl Pts',(-71.0996353689454,5.99985861598442,44.45));
#24313=CARTESIAN_POINT('Ctrl Pts',(-71.099583741031,6.,44.45));
#24314=CARTESIAN_POINT('Ctrl Pts',(-71.1249759611403,0.0004029778460235,
38.5195382755115));
#24315=CARTESIAN_POINT('Ctrl Pts',(-71.124444532618,0.000386110444049271,
38.5180829961864));
#24316=CARTESIAN_POINT('Ctrl Pts',(-71.1227760188122,0.000327740135672606,
38.5135139660428));
#24317=CARTESIAN_POINT('Ctrl Pts',(-71.1158413990602,0.00015687896315957,
38.4945235499686));
#24318=CARTESIAN_POINT('Ctrl Pts',(-71.1102309858307,5.99412278512498E-5,
38.4791587927645));
#24319=CARTESIAN_POINT('Ctrl Pts',(-71.1041805090849,7.89965273412722E-6,
38.462588711091));
#24320=CARTESIAN_POINT('Ctrl Pts',(-71.1006150014995,-2.20980597269683E-7,
38.4528241478644));
#24321=CARTESIAN_POINT('Ctrl Pts',(-71.0999380484808,2.22118770383862E-15,
38.4509702776222));
#24322=CARTESIAN_POINT('Ctrl Pts',(-71.099583741031,2.22044604925032E-15,
38.45));
#24323=CARTESIAN_POINT('Ctrl Pts',(-71.2498342289178,0.00766025837801554,
38.4739453499121));
#24324=CARTESIAN_POINT('Ctrl Pts',(-71.2481873474268,0.00757270113481584,
38.4693721648531));
#24325=CARTESIAN_POINT('Ctrl Pts',(-71.2417364154876,0.00689152341476491,
38.4515647287784));
#24326=CARTESIAN_POINT('Ctrl Pts',(-71.2226921830148,0.00496933901996202,
38.3991367663831));
#24327=CARTESIAN_POINT('Ctrl Pts',(-71.2027396366171,0.00276041256014256,
38.344204338792));
#24328=CARTESIAN_POINT('Ctrl Pts',(-71.1853003558039,0.00110280150098152,
38.2962243229244));
#24329=CARTESIAN_POINT('Ctrl Pts',(-71.1746388922473,0.000211812862022938,
38.2668856359242));
#24330=CARTESIAN_POINT('Ctrl Pts',(-71.1716639991687,1.6754385265044E-15,
38.2586896296946));
#24331=CARTESIAN_POINT('Ctrl Pts',(-71.170555827354,1.66533453693774E-15,
38.2556349368385));
#24332=CARTESIAN_POINT('Ctrl Pts',(-71.3746924966954,0.0149175389100076,
38.4283524243128));
#24333=CARTESIAN_POINT('Ctrl Pts',(-71.371937394986,0.0145270878443996,
38.4206441795261));
#24334=CARTESIAN_POINT('Ctrl Pts',(-71.3644084675142,0.0124921902170271,
38.3999589890528));
#24335=CARTESIAN_POINT('Ctrl Pts',(-71.324903971772,0.00738822179550698,
38.2925712237683));
#24336=CARTESIAN_POINT('Ctrl Pts',(-71.2979963987338,0.00314156754525118,
38.2182024699665));
#24337=CARTESIAN_POINT('Ctrl Pts',(-71.2648879335367,0.00103199899133368,
38.1267307277737));
#24338=CARTESIAN_POINT('Ctrl Pts',(-71.2459709487275,0.000409937861924508,
38.0738533311077));
#24339=CARTESIAN_POINT('Ctrl Pts',(-71.2433899498565,1.12967778653699E-15,
38.0664089817669));
#24340=CARTESIAN_POINT('Ctrl Pts',(-71.241527913677,1.11022302462517E-15,
38.061269873677));
#24341=CARTESIAN_POINT('Ctrl Pts',(-71.4995507644729,0.0221748194419996,
38.3827594987134));
#24342=CARTESIAN_POINT('Ctrl Pts',(-71.4957111847133,0.0212514804357046,
38.3719446037416));
#24343=CARTESIAN_POINT('Ctrl Pts',(-71.4837469740861,0.0180702925442068,
38.3380317230716));
#24344=CARTESIAN_POINT('Ctrl Pts',(-71.4332256595967,0.0086982168980208,
38.1972090149586));
#24345=CARTESIAN_POINT('Ctrl Pts',(-71.3916700903166,0.0033151901126488,
38.0832652396396));
#24346=CARTESIAN_POINT('Ctrl Pts',(-71.346630963495,0.000434975552779805,
37.9603739181246));
#24347=CARTESIAN_POINT('Ctrl Pts',(-71.3201257651823,-1.2100809912375E-5,
37.8879164256937));
#24348=CARTESIAN_POINT('Ctrl Pts',(-71.3151159005443,5.83926949252806E-16,
37.8741283338393));
#24349=CARTESIAN_POINT('Ctrl Pts',(-71.3125,5.55111512312588E-16,37.8669048105155));
#24350=CARTESIAN_POINT('',(-71.1249759611403,0.0004029778460235,38.5195382755115));
#24351=CARTESIAN_POINT('Ctrl Pts',(-71.099583741031,1.77635683940025E-15,
38.45));
#24352=CARTESIAN_POINT('Ctrl Pts',(-71.0997076102035,1.77661612872688E-15,
38.4503392180609));
#24353=CARTESIAN_POINT('Ctrl Pts',(-71.0998330879728,2.29080306181617E-8,
38.450682841484));
#24354=CARTESIAN_POINT('Ctrl Pts',(-71.0999928315323,1.04590663241311E-7,
38.4511203070689));
#24355=CARTESIAN_POINT('Ctrl Pts',(-71.1001600092189,1.90074632695941E-7,
38.4515781313762));
#24356=CARTESIAN_POINT('Ctrl Pts',(-71.1003645763203,3.3899157853453E-7,
38.4521383523869));
#24357=CARTESIAN_POINT('Ctrl Pts',(-71.1006239759305,6.7627716049401E-7,
38.4528487410268));
#24358=CARTESIAN_POINT('Ctrl Pts',(-71.1009173990762,1.05780200688234E-6,
38.4536523061101));
#24359=CARTESIAN_POINT('Ctrl Pts',(-71.1012809729212,1.68218510490073E-6,
38.4546479901747));
#24360=CARTESIAN_POINT('Ctrl Pts',(-71.1017157284715,2.84078832457624E-6,
38.4558386172851));
#24361=CARTESIAN_POINT('Ctrl Pts',(-71.1021914073984,4.10845043020003E-6,
38.4571413176782));
#24362=CARTESIAN_POINT('Ctrl Pts',(-71.1027518533756,6.03043021784941E-6,
38.4586761669085));
#24363=CARTESIAN_POINT('Ctrl Pts',(-71.1033748256032,8.98260865955791E-6,
38.460382255208));
#24364=CARTESIAN_POINT('Ctrl Pts',(-71.1043065151251,1.33977552724482E-5,
38.4629338048942));
#24365=CARTESIAN_POINT('Ctrl Pts',(-71.105376376433,2.02240544760204E-5,
38.4658637623008));
#24366=CARTESIAN_POINT('Ctrl Pts',(-71.1064700237766,2.96381289164316E-5,
38.4688588618043));
#24367=CARTESIAN_POINT('Ctrl Pts',(-71.1072075567534,3.59867845290267E-5,
38.4708786944914));
#24368=CARTESIAN_POINT('Ctrl Pts',(-71.1079547964485,4.34635710976436E-5,
38.4729251106455));
#24369=CARTESIAN_POINT('Ctrl Pts',(-71.1086850574781,5.17716371906118E-5,
38.4749250268998));
#24370=CARTESIAN_POINT('Ctrl Pts',(-71.1093213961134,5.90111628197922E-5,
38.4766677242757));
#24371=CARTESIAN_POINT('Ctrl Pts',(-71.1099446007745,6.68631518634855E-5,
38.4783744513726));
#24372=CARTESIAN_POINT('Ctrl Pts',(-71.1105507959654,7.51735352766403E-5,
38.4800345929261));
#24373=CARTESIAN_POINT('Ctrl Pts',(-71.1111177706792,8.29462417053621E-5,
38.4815873242844));
#24374=CARTESIAN_POINT('Ctrl Pts',(-71.1116696768522,9.11060770996762E-5,
38.4830987860171));
#24375=CARTESIAN_POINT('Ctrl Pts',(-71.1122192145514,9.97858257232309E-5,
38.4846037563199));
#24376=CARTESIAN_POINT('Ctrl Pts',(-71.1127696572181,0.000108479867978652,
38.4861112049768));
#24377=CARTESIAN_POINT('Ctrl Pts',(-71.113320820801,0.000117743551170355,
38.4876206225949));
#24378=CARTESIAN_POINT('Ctrl Pts',(-71.1138867931674,0.000127862606890794,
38.4891705876114));
#24379=CARTESIAN_POINT('Ctrl Pts',(-71.1144995295096,0.000138817758693007,
38.4908486198817));
#24380=CARTESIAN_POINT('Ctrl Pts',(-71.1151294409423,0.000150785770098267,
38.4925736784895));
#24381=CARTESIAN_POINT('Ctrl Pts',(-71.1157735478178,0.000163820814120363,
38.4943376017864));
#24382=CARTESIAN_POINT('Ctrl Pts',(-71.116526402741,0.000179056635129902,
38.4963993377944));
#24383=CARTESIAN_POINT('Ctrl Pts',(-71.1172983542978,0.000195768933336022,
38.4985133567003));
#24384=CARTESIAN_POINT('Ctrl Pts',(-71.1180605344228,0.000213372206193441,
38.5006006022355));
#24385=CARTESIAN_POINT('Ctrl Pts',(-71.118975496028,0.000234504112240295,
38.5031062429141));
#24386=CARTESIAN_POINT('Ctrl Pts',(-71.119874756806,0.000256914198905863,
38.5055688658886));
#24387=CARTESIAN_POINT('Ctrl Pts',(-71.1206908040971,0.00027844441951963,
38.5078035942042));
#24388=CARTESIAN_POINT('Ctrl Pts',(-71.1213197930097,0.000295039376942754,
38.5095260670908));
#24389=CARTESIAN_POINT('Ctrl Pts',(-71.1218985581243,0.000311061768656351,
38.5111109938185));
#24390=CARTESIAN_POINT('Ctrl Pts',(-71.1224030865798,0.000325452800995052,
38.5124926211035));
#24391=CARTESIAN_POINT('Ctrl Pts',(-71.1228613842659,0.000338525159449124,
38.5137476476155));
#24392=CARTESIAN_POINT('Ctrl Pts',(-71.1232581076796,0.000350230036839969,
38.5148340512162));
#24393=CARTESIAN_POINT('Ctrl Pts',(-71.1235880417374,0.000360129646756135,
38.5157375544699));
#24394=CARTESIAN_POINT('Ctrl Pts',(-71.1238976320008,0.000369418844912552,
38.5165853475476));
#24395=CARTESIAN_POINT('Ctrl Pts',(-71.1241482141858,0.000377107971252698,
38.5172715491176));
#24396=CARTESIAN_POINT('Ctrl Pts',(-71.1243508231998,0.000383380394748833,
38.5178263795026));
#24397=CARTESIAN_POINT('Ctrl Pts',(-71.1245404160348,0.000389249859931833,
38.5183455660067));
#24398=CARTESIAN_POINT('Ctrl Pts',(-71.1246879159046,0.000393876624393683,
38.5187494838655));
#24399=CARTESIAN_POINT('Ctrl Pts',(-71.1248181352022,0.000397984060214185,
38.5191060802768));
#24400=CARTESIAN_POINT('Ctrl Pts',(-71.1248726423429,0.000399703349027781,
38.5192553442575));
#24401=CARTESIAN_POINT('Ctrl Pts',(-71.1249243271121,0.000401338995505559,
38.5193968793866));
#24402=CARTESIAN_POINT('Ctrl Pts',(-71.1249759611403,0.000402977846023944,
38.5195382755115));
#24403=CARTESIAN_POINT('Ctrl Pts',(-71.4995507644729,0.0221748194419996,
38.3827594987134));
#24404=CARTESIAN_POINT('Ctrl Pts',(-71.3746924966954,0.0149175389100076,
38.4283524243128));
#24405=CARTESIAN_POINT('Ctrl Pts',(-71.2498342289178,0.00766025837801554,
38.4739453499121));
#24406=CARTESIAN_POINT('Ctrl Pts',(-71.1249759611403,0.0004029778460235,
38.5195382755115));
#24407=CARTESIAN_POINT('Ctrl Pts',(-71.4995507644729,0.0221748194419993,
38.3827594987134));
#24408=CARTESIAN_POINT('Ctrl Pts',(-71.8031180421414,0.095176430570246,
39.2378135490065));
#24409=CARTESIAN_POINT('Ctrl Pts',(-72.1125000002033,0.389138386673939,
40.2118328742239));
#24410=CARTESIAN_POINT('Ctrl Pts',(-72.1125,0.800000000395795,41.0213168380085));
#24411=CARTESIAN_POINT('Ctrl Pts',(-71.3746924966954,0.0149175389100074,
38.4283524243128));
#24412=CARTESIAN_POINT('Ctrl Pts',(-71.6811443918608,0.0668885519346187,
39.283386933046));
#24413=CARTESIAN_POINT('Ctrl Pts',(-72.0098408305469,0.338541460012493,
40.2544419479763));
#24414=CARTESIAN_POINT('Ctrl Pts',(-72.0395269177012,0.74382707347345,41.0573334705988));
#24415=CARTESIAN_POINT('Ctrl Pts',(-71.2498342289178,0.00766025837801544,
38.4739453499121));
#24416=CARTESIAN_POINT('Ctrl Pts',(-71.5591707415801,0.0386006732989913,
39.3289603170856));
#24417=CARTESIAN_POINT('Ctrl Pts',(-71.9071816608906,0.287944533351047,
40.2970510217287));
#24418=CARTESIAN_POINT('Ctrl Pts',(-71.9665538354024,0.687654146551106,
41.0933501031891));
#24419=CARTESIAN_POINT('Ctrl Pts',(-71.1249759611403,0.0004029778460235,
38.5195382755115));
#24420=CARTESIAN_POINT('Ctrl Pts',(-71.4371970912995,0.010312794663364,
39.3745337011251));
#24421=CARTESIAN_POINT('Ctrl Pts',(-71.8045224912342,0.2373476066896,40.3396600954811));
#24422=CARTESIAN_POINT('Ctrl Pts',(-71.8935807531036,0.631481219628762,
41.1293667357794));
#24423=CARTESIAN_POINT('',(-71.8935807531036,0.631481219628701,41.1293667357793));
#24424=CARTESIAN_POINT('Ctrl Pts',(-71.1249759611403,0.0004029778460235,
38.5195382755115));
#24425=CARTESIAN_POINT('Ctrl Pts',(-71.4371970912995,0.010312794663364,
39.3745337011251));
#24426=CARTESIAN_POINT('Ctrl Pts',(-71.8045224912342,0.2373476066896,40.3396600954811));
#24427=CARTESIAN_POINT('Ctrl Pts',(-71.8935807531036,0.631481219628762,
41.1293667357794));
#24428=CARTESIAN_POINT('',(-71.8935807531036,0.631481219628701,41.1293667357793));
#24429=CARTESIAN_POINT('Origin',(-72.0125,6.00000000000001,38.45));
#24430=CARTESIAN_POINT('',(-71.9125,3.00667409058085,43.65));
#24431=CARTESIAN_POINT('',(-72.1125,3.10645162089482,43.4766666666667));
#24432=CARTESIAN_POINT('',(-71.9125,3.00667409058085,43.65));
#24433=CARTESIAN_POINT('',(-72.1125,0.973333333333333,41.3435483791052));
#24434=CARTESIAN_POINT('Origin',(-72.1125,6.00000000000001,38.45));
#24435=CARTESIAN_POINT('',(-71.9125,0.800000000000003,41.4433259094192));
#24436=CARTESIAN_POINT('',(-72.1125,0.973333333333333,41.3435483791052));
#24437=CARTESIAN_POINT('Origin',(-71.9125,6.00000000000001,38.45));
#24438=CARTESIAN_POINT('Ctrl Pts',(-72.1125,0.80000000039573,41.0213168380084));
#24439=CARTESIAN_POINT('Ctrl Pts',(-72.1125,0.856168534250961,41.1319806866355));
#24440=CARTESIAN_POINT('Ctrl Pts',(-72.1125,0.913326151321779,41.2393040181827));
#24441=CARTESIAN_POINT('Ctrl Pts',(-72.1125,0.973333333333339,41.3435483791052));
#24442=CARTESIAN_POINT('Ctrl Pts',(-72.0395269177012,0.743827073473387,
41.0573334705987));
#24443=CARTESIAN_POINT('Ctrl Pts',(-72.0435852768747,0.799233317184012,
41.1670960723289));
#24444=CARTESIAN_POINT('Ctrl Pts',(-72.0458333333333,0.85614614623837,41.2736016445264));
#24445=CARTESIAN_POINT('Ctrl Pts',(-72.0458333333333,0.915555555555561,
41.3768075558765));
#24446=CARTESIAN_POINT('Ctrl Pts',(-71.9665538354024,0.687654146551043,
41.093350103189));
#24447=CARTESIAN_POINT('Ctrl Pts',(-71.9746705537493,0.742298100117063,
41.2022114580222));
#24448=CARTESIAN_POINT('Ctrl Pts',(-71.9791666666667,0.798966141154961,
41.3078992708702));
#24449=CARTESIAN_POINT('Ctrl Pts',(-71.9791666666667,0.857777777777783,
41.4100667326478));
#24450=CARTESIAN_POINT('Ctrl Pts',(-71.8935807531036,0.631481219628699,
41.1293667357793));
#24451=CARTESIAN_POINT('Ctrl Pts',(-71.905755830624,0.685362883050115,41.2373268437155));
#24452=CARTESIAN_POINT('Ctrl Pts',(-71.9125,0.741786136071552,41.3421968972139));
#24453=CARTESIAN_POINT('Ctrl Pts',(-71.9125,0.800000000000005,41.4433259094192));
#24454=CARTESIAN_POINT('Ctrl Pts',(-72.1125,0.973333333333339,41.3435483791052));
#24455=CARTESIAN_POINT('Ctrl Pts',(-72.1125,0.913326151321779,41.2393040181827));
#24456=CARTESIAN_POINT('Ctrl Pts',(-72.1125,0.856168534250961,41.1319806866355));
#24457=CARTESIAN_POINT('Ctrl Pts',(-72.1125,0.80000000039573,41.0213168380084));
#24458=CARTESIAN_POINT('Ctrl Pts',(-71.8935807531036,0.631481219628699,
41.1293667357793));
#24459=CARTESIAN_POINT('Ctrl Pts',(-71.905755830624,0.685362883050115,41.2373268437155));
#24460=CARTESIAN_POINT('Ctrl Pts',(-71.9125,0.741786136071552,41.3421968972139));
#24461=CARTESIAN_POINT('Ctrl Pts',(-71.9125,0.800000000000005,41.4433259094192));
#24462=CARTESIAN_POINT('Ctrl Pts',(-72.1125,3.42868316199152,43.6499999996042));
#24463=CARTESIAN_POINT('Ctrl Pts',(-72.1125000002033,4.23816756991044,44.0608618387509));
#24464=CARTESIAN_POINT('Ctrl Pts',(-71.8031170174309,5.21218945423946,44.3548240219809));
#24465=CARTESIAN_POINT('Ctrl Pts',(-71.4995502651833,6.0672419076457,44.4278253006266));
#24466=CARTESIAN_POINT('Ctrl Pts',(-72.0395269177012,3.3926665294012,43.7061729265265));
#24467=CARTESIAN_POINT('Ctrl Pts',(-72.0098408142592,4.19555849254101,44.111458762353));
#24468=CARTESIAN_POINT('Ctrl Pts',(-71.6811438122403,5.16661477993893,44.3831118133254));
#24469=CARTESIAN_POINT('Ctrl Pts',(-71.3746919924044,6.0216489827177,44.4350825465769));
#24470=CARTESIAN_POINT('Ctrl Pts',(-71.9665538354024,3.35664989681089,43.7623458534489));
#24471=CARTESIAN_POINT('Ctrl Pts',(-71.9071816283152,4.15294941517159,44.1620556859551));
#24472=CARTESIAN_POINT('Ctrl Pts',(-71.5591706070498,5.12104010563839,44.4113996046699));
#24473=CARTESIAN_POINT('Ctrl Pts',(-71.2498337196255,5.9760560577897,44.4423397925272));
#24474=CARTESIAN_POINT('Ctrl Pts',(-71.8935807531036,3.32063326422057,43.8185187803712));
#24475=CARTESIAN_POINT('Ctrl Pts',(-71.8045224423712,4.11034033780217,44.2126526095572));
#24476=CARTESIAN_POINT('Ctrl Pts',(-71.4371974018592,5.07546543133786,44.4396873960144));
#24477=CARTESIAN_POINT('Ctrl Pts',(-71.1249754468465,5.93046313286171,44.4495970384775));
#24478=CARTESIAN_POINT('',(-72.1125,3.42868316190267,43.6499999997796));
#24479=CARTESIAN_POINT('Ctrl Pts',(-71.4995502651833,6.0672419076457,44.4278253006266));
#24480=CARTESIAN_POINT('Ctrl Pts',(-71.8031170174309,5.21218945423946,44.3548240219809));
#24481=CARTESIAN_POINT('Ctrl Pts',(-72.1125000002033,4.23816756991044,44.0608618387509));
#24482=CARTESIAN_POINT('Ctrl Pts',(-72.1125,3.42868316199152,43.6499999996042));
#24483=CARTESIAN_POINT('',(-71.8935807531036,3.32063326422069,43.8185187803713));
#24484=CARTESIAN_POINT('',(-72.1125,3.42868316190267,43.6499999997796));
#24485=CARTESIAN_POINT('Ctrl Pts',(-71.8935807531036,3.32063326422057,43.8185187803712));
#24486=CARTESIAN_POINT('Ctrl Pts',(-71.8045224423712,4.11034033780217,44.2126526095572));
#24487=CARTESIAN_POINT('Ctrl Pts',(-71.4371974018592,5.07546543133786,44.4396873960144));
#24488=CARTESIAN_POINT('Ctrl Pts',(-71.1249754468465,5.93046313286171,44.4495970384775));
#24489=CARTESIAN_POINT('Ctrl Pts',(-72.1125,3.10645162089483,43.4766666666667));
#24490=CARTESIAN_POINT('Ctrl Pts',(-72.1125,3.2106959818173,43.5366738486782));
#24491=CARTESIAN_POINT('Ctrl Pts',(-72.1125,3.31801931336448,43.593831465749));
#24492=CARTESIAN_POINT('Ctrl Pts',(-72.1125,3.42868316199164,43.6499999996043));
#24493=CARTESIAN_POINT('Ctrl Pts',(-72.0458333333333,3.0731924441235,43.5344444444444));
#24494=CARTESIAN_POINT('Ctrl Pts',(-72.0458333333333,3.17639835547357,43.5938538537616));
#24495=CARTESIAN_POINT('Ctrl Pts',(-72.0435852768747,3.28290392767114,43.650766682816));
#24496=CARTESIAN_POINT('Ctrl Pts',(-72.0395269177012,3.39266652940132,43.7061729265266));
#24497=CARTESIAN_POINT('Ctrl Pts',(-71.9791666666667,3.03993326735218,43.5922222222222));
#24498=CARTESIAN_POINT('Ctrl Pts',(-71.9791666666667,3.14210072912984,43.651033858845));
#24499=CARTESIAN_POINT('Ctrl Pts',(-71.9746705537493,3.2477885419778,43.7077018998829));
#24500=CARTESIAN_POINT('Ctrl Pts',(-71.9665538354024,3.35664989681101,43.762345853449));
#24501=CARTESIAN_POINT('Ctrl Pts',(-71.9125,3.00667409058085,43.65));
#24502=CARTESIAN_POINT('Ctrl Pts',(-71.9125,3.1078031027861,43.7082138639284));
#24503=CARTESIAN_POINT('Ctrl Pts',(-71.905755830624,3.21267315628445,43.7646371169499));
#24504=CARTESIAN_POINT('Ctrl Pts',(-71.8935807531036,3.32063326422069,43.8185187803713));
#24505=CARTESIAN_POINT('Ctrl Pts',(-72.1125,3.42868316199164,43.6499999996043));
#24506=CARTESIAN_POINT('Ctrl Pts',(-72.1125,3.31801931336448,43.593831465749));
#24507=CARTESIAN_POINT('Ctrl Pts',(-72.1125,3.2106959818173,43.5366738486782));
#24508=CARTESIAN_POINT('Ctrl Pts',(-72.1125,3.10645162089483,43.4766666666667));
#24509=CARTESIAN_POINT('Ctrl Pts',(-71.9125,3.00667409058085,43.65));
#24510=CARTESIAN_POINT('Ctrl Pts',(-71.9125,3.1078031027861,43.7082138639284));
#24511=CARTESIAN_POINT('Ctrl Pts',(-71.905755830624,3.21267315628445,43.7646371169499));
#24512=CARTESIAN_POINT('Ctrl Pts',(-71.8935807531036,3.32063326422069,43.8185187803713));
#24513=CARTESIAN_POINT('Origin',(-72.1125,63.5,-31.75));
#24514=CARTESIAN_POINT('',(-72.1125,123.993325909419,43.65));
#24515=CARTESIAN_POINT('',(-72.1125,34.75,43.65));
#24516=CARTESIAN_POINT('',(-72.1125,126.2,41.4433259094192));
#24517=CARTESIAN_POINT('Origin',(-72.1125,121.,38.45));
#24518=CARTESIAN_POINT('',(-72.1125,126.2,-104.943325909419));
#24519=CARTESIAN_POINT('',(-72.1125,126.2,3.35000000000001));
#24520=CARTESIAN_POINT('',(-72.1125,123.993325909419,-107.15));
#24521=CARTESIAN_POINT('Origin',(-72.1125,121.,-101.95));
#24522=CARTESIAN_POINT('',(-72.1125,92.25,-107.15));
#24523=CARTESIAN_POINT('Origin',(-67.35,6.00000000000001,38.45));
#24524=CARTESIAN_POINT('Origin',(-68.15,0.800000000000001,-66.85));
#24525=CARTESIAN_POINT('Origin',(-71.3125,34.75,43.65));
#24526=CARTESIAN_POINT('Ctrl Pts',(-71.3125,121.,44.45));
#24527=CARTESIAN_POINT('Ctrl Pts',(-71.4899908431149,121.486078692623,44.45));
#24528=CARTESIAN_POINT('Ctrl Pts',(-71.6844866658569,122.014025751789,44.387608349819));
#24529=CARTESIAN_POINT('Ctrl Pts',(-71.9943880775948,123.043713064318,44.1162803662604));
#24530=CARTESIAN_POINT('Ctrl Pts',(-72.1125,123.544851663295,43.9081595347366));
#24531=CARTESIAN_POINT('Ctrl Pts',(-72.1125,123.993325909419,43.65));
#24532=CARTESIAN_POINT('Origin',(-67.35,121.,38.45));
#24533=CARTESIAN_POINT('',(-68.15,127.,38.45));
#24534=CARTESIAN_POINT('Ctrl Pts',(-68.15,127.,38.45));
#24535=CARTESIAN_POINT('Ctrl Pts',(-67.9725091568851,127.,38.9360786926232));
#24536=CARTESIAN_POINT('Ctrl Pts',(-67.7780133341431,126.937608349819,39.4640257517887));
#24537=CARTESIAN_POINT('Ctrl Pts',(-67.4681119224052,126.66628036626,40.4937130643181));
#24538=CARTESIAN_POINT('Ctrl Pts',(-67.35,126.458159534737,40.9948516632952));
#24539=CARTESIAN_POINT('Ctrl Pts',(-67.35,126.2,41.4433259094192));
#24540=CARTESIAN_POINT('',(-71.3125,127.,38.45));
#24541=CARTESIAN_POINT('',(-67.35,127.,38.45));
#24542=CARTESIAN_POINT('Ctrl Pts',(-72.1125,126.2,41.4433259094192));
#24543=CARTESIAN_POINT('Ctrl Pts',(-72.1125,126.458159534737,40.9948516632952));
#24544=CARTESIAN_POINT('Ctrl Pts',(-71.9943880775948,126.66628036626,40.4937130643181));
#24545=CARTESIAN_POINT('Ctrl Pts',(-71.6844866658569,126.937608349819,39.4640257517887));
#24546=CARTESIAN_POINT('Ctrl Pts',(-71.4899908431149,127.,38.9360786926232));
#24547=CARTESIAN_POINT('Ctrl Pts',(-71.3125,127.,38.45));
#24548=CARTESIAN_POINT('Origin',(-71.3125,126.2,3.35000000000001));
#24549=CARTESIAN_POINT('',(-71.3125,127.,-101.95));
#24550=CARTESIAN_POINT('Ctrl Pts',(-71.3125,127.,-101.95));
#24551=CARTESIAN_POINT('Ctrl Pts',(-71.4899908431149,127.,-102.436078692623));
#24552=CARTESIAN_POINT('Ctrl Pts',(-71.6844866658568,126.937608349819,-102.964025751789));
#24553=CARTESIAN_POINT('Ctrl Pts',(-71.9943880775948,126.66628036626,-103.993713064318));
#24554=CARTESIAN_POINT('Ctrl Pts',(-72.1125,126.458159534737,-104.494851663295));
#24555=CARTESIAN_POINT('Ctrl Pts',(-72.1125,126.2,-104.943325909419));
#24556=CARTESIAN_POINT('',(-71.3125,127.,3.35000000000001));
#24557=CARTESIAN_POINT('Origin',(-67.35,121.,-101.95));
#24558=CARTESIAN_POINT('',(-68.15,127.,-101.95));
#24559=CARTESIAN_POINT('',(-67.35,127.,-101.95));
#24560=CARTESIAN_POINT('Ctrl Pts',(-67.35,126.2,-104.943325909419));
#24561=CARTESIAN_POINT('Ctrl Pts',(-67.35,126.458159534737,-104.494851663295));
#24562=CARTESIAN_POINT('Ctrl Pts',(-67.4681119224052,126.66628036626,-103.993713064318));
#24563=CARTESIAN_POINT('Ctrl Pts',(-67.7780133341432,126.937608349819,-102.964025751789));
#24564=CARTESIAN_POINT('Ctrl Pts',(-67.9725091568851,127.,-102.436078692623));
#24565=CARTESIAN_POINT('Ctrl Pts',(-68.15,127.,-101.95));
#24566=CARTESIAN_POINT('Ctrl Pts',(-72.1125,123.993325909419,-107.15));
#24567=CARTESIAN_POINT('Ctrl Pts',(-72.1125,123.544851663295,-107.408159534737));
#24568=CARTESIAN_POINT('Ctrl Pts',(-71.9943880775948,123.043713064318,-107.61628036626));
#24569=CARTESIAN_POINT('Ctrl Pts',(-71.6844866658569,122.014025751789,-107.887608349819));
#24570=CARTESIAN_POINT('Ctrl Pts',(-71.4899908431149,121.486078692623,-107.95));
#24571=CARTESIAN_POINT('Ctrl Pts',(-71.3125,121.,-107.95));
#24572=CARTESIAN_POINT('Origin',(-67.35,127.,38.45));
#24573=CARTESIAN_POINT('',(-68.15,127.,3.35000000000001));
#24574=CARTESIAN_POINT('Origin',(-68.15,126.2,3.35000000000001));
#24575=CARTESIAN_POINT('Origin',(-71.3125,92.25,-107.15));
#32284=UNCERTAINTY_MEASURE_WITH_UNIT(LENGTH_MEASURE(0.01),#32310,
'DISTANCE_ACCURACY_VALUE',
'Maximum model space distance between geometric entities at asserted c
onnectivities');
#32293=UNCERTAINTY_MEASURE_WITH_UNIT(LENGTH_MEASURE(0.01),#32310,
'DISTANCE_ACCURACY_VALUE',
'Maximum model space distance between geometric entities at asserted c
onnectivities');
#32300=(
GEOMETRIC_REPRESENTATION_CONTEXT(3)
GLOBAL_UNCERTAINTY_ASSIGNED_CONTEXT((#32284))
GLOBAL_UNIT_ASSIGNED_CONTEXT((#32310,#32312,#32313))
REPRESENTATION_CONTEXT('','3D')
);
#32309=(
GEOMETRIC_REPRESENTATION_CONTEXT(3)
GLOBAL_UNCERTAINTY_ASSIGNED_CONTEXT((#32293))
GLOBAL_UNIT_ASSIGNED_CONTEXT((#32310,#32312,#32313))
REPRESENTATION_CONTEXT('','3D')
);
#32310=(
LENGTH_UNIT()
NAMED_UNIT(*)
SI_UNIT(.MILLI.,.METRE.)
);
#32312=(
NAMED_UNIT(*)
PLANE_ANGLE_UNIT()
SI_UNIT($,.RADIAN.)
);
#32313=(
NAMED_UNIT(*)
SI_UNIT($,.STERADIAN.)
SOLID_ANGLE_UNIT()
);
#32320=SHAPE_DEFINITION_REPRESENTATION(#32335,#32367);
#32335=PRODUCT_DEFINITION_SHAPE('',$,#32383);
#32367=SHAPE_REPRESENTATION('',(#14378),#32300);
#32376=PRODUCT_DEFINITION_CONTEXT('part definition',#32423,'design');
#32383=PRODUCT_DEFINITION('2026-10-25-00-35-17-554',
'06_Inner_End_Plate_6in',#32398,#32376);
#32398=PRODUCT_DEFINITION_FORMATION('',$,#32431);
#32423=APPLICATION_CONTEXT(
'Core Data for Automotive Mechanical Design Process');
#32424=PRODUCT_CONTEXT('part definition',#32423,'mechanical');
#32431=PRODUCT('2026-10-25-00-35-17-554','06_Inner_End_Plate_6in',$,(#32424));
#32489=COLOUR_RGB('Sky Blue',0.24,0.69,0.87);
#32490=FILL_AREA_STYLE_COLOUR('',#32489);
#32491=FILL_AREA_STYLE('',(#32490));
#32492=SURFACE_STYLE_FILL_AREA(#32491);
#32493=SURFACE_SIDE_STYLE('',(#32492));
#32494=SURFACE_STYLE_USAGE(.BOTH.,#32493);
#32495=PRESENTATION_STYLE_ASSIGNMENT((#32494));
ENDSEC;
END-ISO-10303-21;
